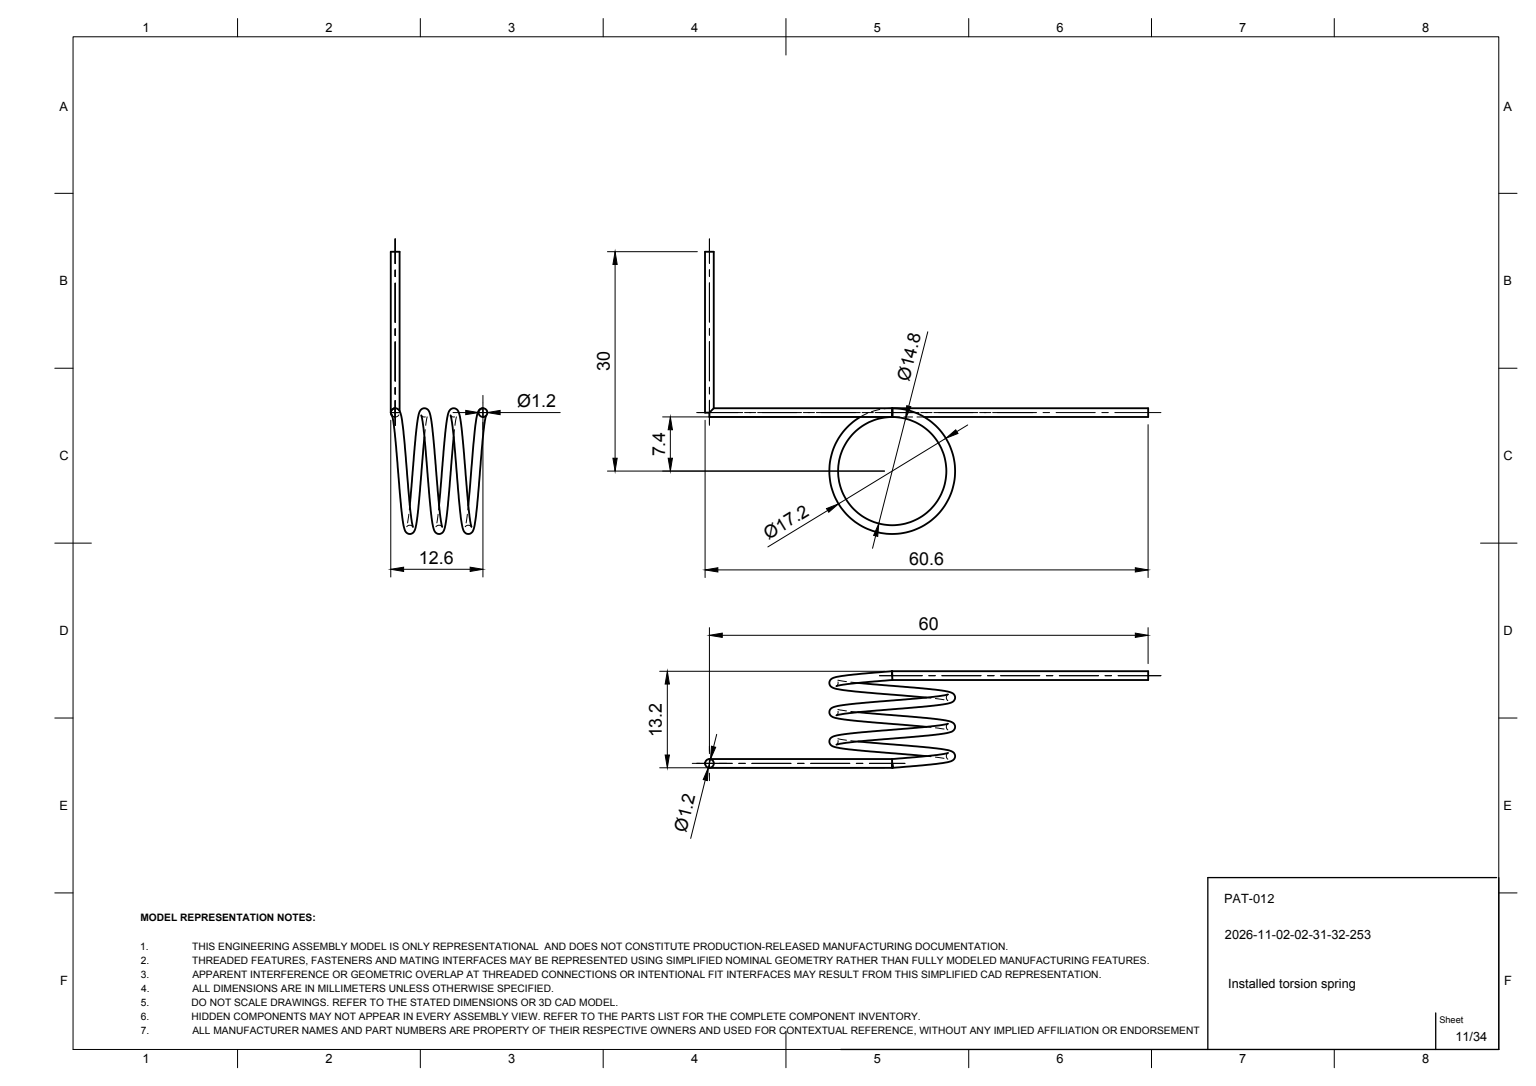
ISO-10303-21;
HEADER;
/* Generated by software containing ST-Developer
 * from STEP Tools, Inc. (www.steptools.com) 
 */

FILE_DESCRIPTION(
/* description */ ('Belt tensioner idler arm'),
/* implementation_level */ '2;1');

FILE_NAME(
/* name */ 'Installed torsion spring.step',
/* time_stamp */ '2026-10-28T03:22:15-07:00',
/* author */ (''),
/* organization */ (''),
/* preprocessor_version */ 'ST-DEVELOPER v20.2',
/* originating_system */ 'Autodesk Translation Framework v15.17.0.0',
/* authorisation */ '');

FILE_SCHEMA (('AUTOMOTIVE_DESIGN { 1 0 10303 214 3 1 1 }'));
ENDSEC;

DATA;
#10=MECHANICAL_DESIGN_GEOMETRIC_PRESENTATION_REPRESENTATION('',(#453),#12779);
#315=B_SPLINE_SURFACE_WITH_KNOTS('',3,3,((#9880,#9881,#9882,#9883,#9884,
#9885,#9886,#9887,#9888,#9889,#9890,#9891,#9892,#9893,#9894,#9895,#9896,
#9897,#9898,#9899,#9900,#9901,#9902,#9903,#9904,#9905,#9906,#9907,#9908,
#9909,#9910,#9911,#9912,#9913,#9914,#9915,#9916,#9917,#9918,#9919,#9920),
(#9921,#9922,#9923,#9924,#9925,#9926,#9927,#9928,#9929,#9930,#9931,#9932,
#9933,#9934,#9935,#9936,#9937,#9938,#9939,#9940,#9941,#9942,#9943,#9944,
#9945,#9946,#9947,#9948,#9949,#9950,#9951,#9952,#9953,#9954,#9955,#9956,
#9957,#9958,#9959,#9960,#9961),(#9962,#9963,#9964,#9965,#9966,#9967,#9968,
#9969,#9970,#9971,#9972,#9973,#9974,#9975,#9976,#9977,#9978,#9979,#9980,
#9981,#9982,#9983,#9984,#9985,#9986,#9987,#9988,#9989,#9990,#9991,#9992,
#9993,#9994,#9995,#9996,#9997,#9998,#9999,#10000,#10001,#10002),(#10003,
#10004,#10005,#10006,#10007,#10008,#10009,#10010,#10011,#10012,#10013,#10014,
#10015,#10016,#10017,#10018,#10019,#10020,#10021,#10022,#10023,#10024,#10025,
#10026,#10027,#10028,#10029,#10030,#10031,#10032,#10033,#10034,#10035,#10036,
#10037,#10038,#10039,#10040,#10041,#10042,#10043),(#10044,#10045,#10046,
#10047,#10048,#10049,#10050,#10051,#10052,#10053,#10054,#10055,#10056,#10057,
#10058,#10059,#10060,#10061,#10062,#10063,#10064,#10065,#10066,#10067,#10068,
#10069,#10070,#10071,#10072,#10073,#10074,#10075,#10076,#10077,#10078,#10079,
#10080,#10081,#10082,#10083,#10084),(#10085,#10086,#10087,#10088,#10089,
#10090,#10091,#10092,#10093,#10094,#10095,#10096,#10097,#10098,#10099,#10100,
#10101,#10102,#10103,#10104,#10105,#10106,#10107,#10108,#10109,#10110,#10111,
#10112,#10113,#10114,#10115,#10116,#10117,#10118,#10119,#10120,#10121,#10122,
#10123,#10124,#10125),(#10126,#10127,#10128,#10129,#10130,#10131,#10132,
#10133,#10134,#10135,#10136,#10137,#10138,#10139,#10140,#10141,#10142,#10143,
#10144,#10145,#10146,#10147,#10148,#10149,#10150,#10151,#10152,#10153,#10154,
#10155,#10156,#10157,#10158,#10159,#10160,#10161,#10162,#10163,#10164,#10165,
#10166),(#10167,#10168,#10169,#10170,#10171,#10172,#10173,#10174,#10175,
#10176,#10177,#10178,#10179,#10180,#10181,#10182,#10183,#10184,#10185,#10186,
#10187,#10188,#10189,#10190,#10191,#10192,#10193,#10194,#10195,#10196,#10197,
#10198,#10199,#10200,#10201,#10202,#10203,#10204,#10205,#10206,#10207),
(#10208,#10209,#10210,#10211,#10212,#10213,#10214,#10215,#10216,#10217,
#10218,#10219,#10220,#10221,#10222,#10223,#10224,#10225,#10226,#10227,#10228,
#10229,#10230,#10231,#10232,#10233,#10234,#10235,#10236,#10237,#10238,#10239,
#10240,#10241,#10242,#10243,#10244,#10245,#10246,#10247,#10248),(#10249,
#10250,#10251,#10252,#10253,#10254,#10255,#10256,#10257,#10258,#10259,#10260,
#10261,#10262,#10263,#10264,#10265,#10266,#10267,#10268,#10269,#10270,#10271,
#10272,#10273,#10274,#10275,#10276,#10277,#10278,#10279,#10280,#10281,#10282,
#10283,#10284,#10285,#10286,#10287,#10288,#10289)),.UNSPECIFIED.,.T.,.F.,
 .F.,(4,1,1,1,1,1,1,4),(4,1,1,1,1,1,1,1,1,1,1,1,1,1,1,1,1,1,1,1,1,1,1,1,
1,1,1,1,1,1,1,1,1,1,1,1,1,1,4),(-3.14159265358988,-2.24399475256421,-1.34639685153853,
-0.448798950512863,0.448798950512809,1.34639685153848,2.24399475256415,
3.14159265358982),(0.,0.0357142857142857,0.0714285714285714,0.107142857142857,
0.125,0.133928571428571,0.142857142857143,0.174603174603175,0.19047619047619,
0.214285714285714,0.238095238095238,0.261904761904762,0.273809523809524,
0.285714285714286,0.30952380952381,0.333333333333333,0.357142857142857,
0.380952380952381,0.412698412698413,0.428571428571429,0.452380952380952,
0.476190476190476,0.5,0.535714285714286,0.571428571428571,0.607142857142857,
0.642857142857143,0.678571428571428,0.714285714285714,0.738095238095238,
0.761904761904762,0.785714285714286,0.809523809523809,0.833333333333333,
0.857142857142857,0.892857142857143,0.928571428571429,0.964285714285714,
1.),.UNSPECIFIED.);
#316=ELLIPSE('',#6695,0.0848528137423855,0.0599999999999996);
#324=B_SPLINE_CURVE_WITH_KNOTS('',3,(#9810,#9811,#9812,#9813,#9814,#9815,
#9816),.UNSPECIFIED.,.F.,.F.,(4,3,4),(-0.00330054689312876,0.,0.00113632995669113),
 .UNSPECIFIED.);
#325=B_SPLINE_CURVE_WITH_KNOTS('',3,(#9817,#9818,#9819,#9820,#9821,#9822,
#9823,#9824,#9825,#9826,#9827,#9828,#9829,#9830,#9831,#9832,#9833,#9834,
#9835,#9836,#9837,#9838,#9839,#9840,#9841,#9842,#9843,#9844,#9845,#9846,
#9847,#9848,#9849,#9850,#9851,#9852,#9853,#9854,#9855,#9856,#9857,#9858,
#9859,#9860,#9861,#9862,#9863,#9864,#9865,#9866,#9867,#9868,#9869,#9870,
#9871,#9872,#9873,#9874),.UNSPECIFIED.,.F.,.F.,(4,3,3,3,3,3,3,3,3,3,3,3,
3,3,3,3,3,3,3,4),(-0.187914936482157,-0.186780639062755,-0.170605853942537,
-0.165437814146277,-0.164113083876462,-0.147906084064185,-0.140662734614346,
-0.124376338567638,-0.117231977811975,-0.111403976662175,-0.095176489596115,
-0.0938100295088016,-0.0774833765802454,-0.070381765801811,-0.0573630234982956,
-0.046936415200375,-0.0306169940923779,-0.0234729466450609,-0.00725345698800663,
-0.00330054689312876),.UNSPECIFIED.);
#326=B_SPLINE_CURVE_WITH_KNOTS('',3,(#10292,#10293,#10294,#10295,#10296,
#10297,#10298,#10299,#10300,#10301,#10302,#10303,#10304,#10305,#10306,#10307,
#10308,#10309,#10310,#10311,#10312,#10313,#10314,#10315,#10316,#10317,#10318,
#10319,#10320,#10321,#10322,#10323,#10324,#10325,#10326,#10327,#10328,#10329,
#10330,#10331,#10332,#10333,#10334,#10335,#10336,#10337,#10338,#10339,#10340,
#10341,#10342,#10343,#10344,#10345,#10346,#10347,#10348,#10349,#10350,#10351,
#10352),.UNSPECIFIED.,.F.,.F.,(4,3,3,3,3,3,3,3,3,3,3,3,3,3,3,3,3,3,3,3,
4),(-0.187914936422243,-0.186780639028976,-0.174403055129874,-0.164113083856377,
-0.147782436669538,-0.140662734596942,-0.124476652868443,-0.120351214576537,
-0.117231977796532,-0.101004644530292,-0.0938100294949805,-0.0775453096070019,
-0.0703817657897228,-0.0663337540103528,-0.0501165597360029,-0.0469364151905663,
-0.0306116886006247,-0.0234729466383474,-0.0122741858231731,0.,0.00113632996403919),
 .UNSPECIFIED.);
#327=B_SPLINE_CURVE_WITH_KNOTS('',3,(#10356,#10357,#10358,#10359,#10360,
#10361,#10362,#10363,#10364,#10365,#10366,#10367,#10368,#10369,#10370,#10371,
#10372,#10373,#10374,#10375,#10376,#10377,#10378,#10379,#10380,#10381,#10382,
#10383,#10384,#10385,#10386,#10387,#10388,#10389,#10390,#10391,#10392,#10393,
#10394,#10395,#10396),.UNSPECIFIED.,.F.,.F.,(4,1,1,1,1,1,1,1,1,1,1,1,1,
1,1,1,1,1,1,1,1,1,1,1,1,1,1,1,1,1,1,1,1,1,1,1,1,1,4),(0.,0.0357142857142857,
0.0714285714285714,0.107142857142857,0.125,0.133928571428571,0.142857142857143,
0.174603174603175,0.19047619047619,0.214285714285714,0.238095238095238,
0.261904761904762,0.273809523809524,0.285714285714286,0.30952380952381,
0.333333333333333,0.357142857142857,0.380952380952381,0.412698412698413,
0.428571428571429,0.452380952380952,0.476190476190476,0.5,0.535714285714286,
0.571428571428571,0.607142857142857,0.642857142857143,0.678571428571428,
0.714285714285714,0.738095238095238,0.761904761904762,0.785714285714286,
0.809523809523809,0.833333333333333,0.857142857142857,0.892857142857143,
0.928571428571429,0.964285714285714,0.999978445633173),.UNSPECIFIED.);
#328=B_SPLINE_CURVE_WITH_KNOTS('',3,(#10397,#10398,#10399,#10400),
 .UNSPECIFIED.,.F.,.F.,(4,4),(0.999978445544819,0.999989048312129),
 .UNSPECIFIED.);
#385=SHAPE_REPRESENTATION_RELATIONSHIP('SRR','None',#12931,#419);
#419=ADVANCED_BREP_SHAPE_REPRESENTATION('',(#495),#12748);
#453=STYLED_ITEM('',(#13184),#495);
#495=MANIFOLD_SOLID_BREP('Body1',#6187);
#693=PLANE('',#6697);
#694=PLANE('',#6698);
#695=PLANE('',#6699);
#696=PLANE('',#6704);
#697=PLANE('',#6705);
#698=PLANE('',#6712);
#699=PLANE('',#6713);
#700=PLANE('',#6714);
#885=FACE_OUTER_BOUND('',#1278,.T.);
#886=FACE_OUTER_BOUND('',#1279,.T.);
#887=FACE_OUTER_BOUND('',#1280,.T.);
#888=FACE_OUTER_BOUND('',#1281,.T.);
#889=FACE_OUTER_BOUND('',#1282,.T.);
#890=FACE_OUTER_BOUND('',#1283,.T.);
#891=FACE_OUTER_BOUND('',#1284,.T.);
#892=FACE_OUTER_BOUND('',#1285,.T.);
#893=FACE_OUTER_BOUND('',#1286,.T.);
#894=FACE_OUTER_BOUND('',#1287,.T.);
#895=FACE_OUTER_BOUND('',#1288,.T.);
#896=FACE_OUTER_BOUND('',#1289,.T.);
#1278=EDGE_LOOP('',(#4280,#4281,#4282,#4283,#4284));
#1279=EDGE_LOOP('',(#4285));
#1280=EDGE_LOOP('',(#4286,#4287));
#1281=EDGE_LOOP('',(#4288,#4289,#4290));
#1282=EDGE_LOOP('',(#4291,#4292,#4293,#4294,#4295,#4296,#4297,#4298));
#1283=EDGE_LOOP('',(#4299,#4300));
#1284=EDGE_LOOP('',(#4301,#4302));
#1285=EDGE_LOOP('',(#4303,#4304,#4305,#4306,#4307,#4308,#4309,#4310,#4311,
#4312));
#1286=EDGE_LOOP('',(#4313,#4314,#4315,#4316,#4317));
#1287=EDGE_LOOP('',(#4318,#4319));
#1288=EDGE_LOOP('',(#4320));
#1289=EDGE_LOOP('',(#4321,#4322,#4323));
#1763=LINE('',#9794,#2112);
#1764=LINE('',#9800,#2113);
#1765=LINE('',#9875,#2114);
#1766=LINE('',#9877,#2115);
#1767=LINE('',#10405,#2116);
#1768=LINE('',#10408,#2117);
#2112=VECTOR('',#7675,0.0599999999999996);
#2113=VECTOR('',#7684,1.);
#2114=VECTOR('',#7695,0.0600000000000001);
#2115=VECTOR('',#7698,1.);
#2116=VECTOR('',#7711,0.06);
#2117=VECTOR('',#7716,1.);
#2439=CIRCLE('',#6694,0.0599999999999996);
#2440=CIRCLE('',#6696,0.0599999999999996);
#2441=CIRCLE('',#6700,0.0600000000000001);
#2442=CIRCLE('',#6701,0.0600000000000001);
#2443=CIRCLE('',#6703,0.0600000000000001);
#2444=CIRCLE('',#6706,0.06);
#2445=CIRCLE('',#6707,0.06);
#2446=CIRCLE('',#6708,0.06);
#2447=CIRCLE('',#6710,0.0600000000000001);
#2448=CIRCLE('',#6711,0.0600000000000001);
#2834=VERTEX_POINT('',#9791);
#2835=VERTEX_POINT('',#9793);
#2836=VERTEX_POINT('',#9795);
#2837=VERTEX_POINT('',#9802);
#2838=VERTEX_POINT('',#9806);
#2839=VERTEX_POINT('',#9807);
#2840=VERTEX_POINT('',#9809);
#2841=VERTEX_POINT('',#10290);
#2842=VERTEX_POINT('',#10291);
#2843=VERTEX_POINT('',#10353);
#2844=VERTEX_POINT('',#10355);
#2845=VERTEX_POINT('',#10404);
#3395=EDGE_CURVE('',#2834,#2834,#2439,.T.);
#3396=EDGE_CURVE('',#2834,#2835,#1763,.T.);
#3397=EDGE_CURVE('',#2836,#2835,#316,.T.);
#3398=EDGE_CURVE('',#2836,#2835,#2440,.T.);
#3399=EDGE_CURVE('',#2835,#2836,#1764,.T.);
#3400=EDGE_CURVE('',#2836,#2837,#2441,.T.);
#3401=EDGE_CURVE('',#2837,#2835,#2442,.T.);
#3402=EDGE_CURVE('',#2838,#2839,#2443,.T.);
#3403=EDGE_CURVE('',#2840,#2839,#324,.T.);
#3404=EDGE_CURVE('',#2838,#2840,#325,.T.);
#3405=EDGE_CURVE('',#2837,#2838,#1765,.T.);
#3406=EDGE_CURVE('',#2839,#2838,#1766,.T.);
#3407=EDGE_CURVE('',#2838,#2839,#2444,.T.);
#3408=EDGE_CURVE('',#2841,#2842,#326,.T.);
#3409=EDGE_CURVE('',#2842,#2843,#2445,.T.);
#3410=EDGE_CURVE('',#2843,#2844,#327,.T.);
#3411=EDGE_CURVE('',#2844,#2840,#328,.T.);
#3412=EDGE_CURVE('',#2843,#2841,#2446,.T.);
#3413=EDGE_CURVE('',#2842,#2841,#2447,.T.);
#3414=EDGE_CURVE('',#2841,#2845,#1767,.T.);
#3415=EDGE_CURVE('',#2845,#2845,#2448,.T.);
#3416=EDGE_CURVE('',#2842,#2841,#1768,.T.);
#4280=ORIENTED_EDGE('',*,*,#3395,.F.);
#4281=ORIENTED_EDGE('',*,*,#3396,.T.);
#4282=ORIENTED_EDGE('',*,*,#3397,.F.);
#4283=ORIENTED_EDGE('',*,*,#3398,.T.);
#4284=ORIENTED_EDGE('',*,*,#3396,.F.);
#4285=ORIENTED_EDGE('',*,*,#3395,.T.);
#4286=ORIENTED_EDGE('',*,*,#3399,.F.);
#4287=ORIENTED_EDGE('',*,*,#3398,.F.);
#4288=ORIENTED_EDGE('',*,*,#3399,.T.);
#4289=ORIENTED_EDGE('',*,*,#3400,.T.);
#4290=ORIENTED_EDGE('',*,*,#3401,.T.);
#4291=ORIENTED_EDGE('',*,*,#3402,.T.);
#4292=ORIENTED_EDGE('',*,*,#3403,.F.);
#4293=ORIENTED_EDGE('',*,*,#3404,.F.);
#4294=ORIENTED_EDGE('',*,*,#3405,.F.);
#4295=ORIENTED_EDGE('',*,*,#3400,.F.);
#4296=ORIENTED_EDGE('',*,*,#3397,.T.);
#4297=ORIENTED_EDGE('',*,*,#3401,.F.);
#4298=ORIENTED_EDGE('',*,*,#3405,.T.);
#4299=ORIENTED_EDGE('',*,*,#3406,.F.);
#4300=ORIENTED_EDGE('',*,*,#3402,.F.);
#4301=ORIENTED_EDGE('',*,*,#3406,.T.);
#4302=ORIENTED_EDGE('',*,*,#3407,.T.);
#4303=ORIENTED_EDGE('',*,*,#3408,.T.);
#4304=ORIENTED_EDGE('',*,*,#3409,.T.);
#4305=ORIENTED_EDGE('',*,*,#3410,.T.);
#4306=ORIENTED_EDGE('',*,*,#3411,.T.);
#4307=ORIENTED_EDGE('',*,*,#3403,.T.);
#4308=ORIENTED_EDGE('',*,*,#3407,.F.);
#4309=ORIENTED_EDGE('',*,*,#3404,.T.);
#4310=ORIENTED_EDGE('',*,*,#3411,.F.);
#4311=ORIENTED_EDGE('',*,*,#3410,.F.);
#4312=ORIENTED_EDGE('',*,*,#3412,.T.);
#4313=ORIENTED_EDGE('',*,*,#3413,.F.);
#4314=ORIENTED_EDGE('',*,*,#3408,.F.);
#4315=ORIENTED_EDGE('',*,*,#3414,.T.);
#4316=ORIENTED_EDGE('',*,*,#3415,.T.);
#4317=ORIENTED_EDGE('',*,*,#3414,.F.);
#4318=ORIENTED_EDGE('',*,*,#3416,.F.);
#4319=ORIENTED_EDGE('',*,*,#3413,.T.);
#4320=ORIENTED_EDGE('',*,*,#3415,.F.);
#4321=ORIENTED_EDGE('',*,*,#3416,.T.);
#4322=ORIENTED_EDGE('',*,*,#3412,.F.);
#4323=ORIENTED_EDGE('',*,*,#3409,.F.);
#5680=CYLINDRICAL_SURFACE('',#6693,0.0599999999999996);
#5681=CYLINDRICAL_SURFACE('',#6702,0.0600000000000001);
#5682=CYLINDRICAL_SURFACE('',#6709,0.0600000000000001);
#5862=ADVANCED_FACE('',(#885),#5680,.T.);
#5863=ADVANCED_FACE('',(#886),#693,.T.);
#5864=ADVANCED_FACE('',(#887),#694,.F.);
#5865=ADVANCED_FACE('',(#888),#695,.T.);
#5866=ADVANCED_FACE('',(#889),#5681,.T.);
#5867=ADVANCED_FACE('',(#890),#696,.F.);
#5868=ADVANCED_FACE('',(#891),#697,.T.);
#5869=ADVANCED_FACE('',(#892),#315,.T.);
#5870=ADVANCED_FACE('',(#893),#5682,.T.);
#5871=ADVANCED_FACE('',(#894),#698,.T.);
#5872=ADVANCED_FACE('',(#895),#699,.F.);
#5873=ADVANCED_FACE('',(#896),#700,.F.);
#6187=CLOSED_SHELL('',(#5862,#5863,#5864,#5865,#5866,#5867,#5868,#5869,
#5870,#5871,#5872,#5873));
#6692=AXIS2_PLACEMENT_3D('',#9789,#7669,#7670);
#6693=AXIS2_PLACEMENT_3D('',#9790,#7671,#7672);
#6694=AXIS2_PLACEMENT_3D('',#9792,#7673,#7674);
#6695=AXIS2_PLACEMENT_3D('',#9796,#7676,#7677);
#6696=AXIS2_PLACEMENT_3D('',#9797,#7678,#7679);
#6697=AXIS2_PLACEMENT_3D('',#9798,#7680,#7681);
#6698=AXIS2_PLACEMENT_3D('',#9799,#7682,#7683);
#6699=AXIS2_PLACEMENT_3D('',#9801,#7685,#7686);
#6700=AXIS2_PLACEMENT_3D('',#9803,#7687,#7688);
#6701=AXIS2_PLACEMENT_3D('',#9804,#7689,#7690);
#6702=AXIS2_PLACEMENT_3D('',#9805,#7691,#7692);
#6703=AXIS2_PLACEMENT_3D('',#9808,#7693,#7694);
#6704=AXIS2_PLACEMENT_3D('',#9876,#7696,#7697);
#6705=AXIS2_PLACEMENT_3D('',#9878,#7699,#7700);
#6706=AXIS2_PLACEMENT_3D('',#9879,#7701,#7702);
#6707=AXIS2_PLACEMENT_3D('',#10354,#7703,#7704);
#6708=AXIS2_PLACEMENT_3D('',#10401,#7705,#7706);
#6709=AXIS2_PLACEMENT_3D('',#10402,#7707,#7708);
#6710=AXIS2_PLACEMENT_3D('',#10403,#7709,#7710);
#6711=AXIS2_PLACEMENT_3D('',#10406,#7712,#7713);
#6712=AXIS2_PLACEMENT_3D('',#10407,#7714,#7715);
#6713=AXIS2_PLACEMENT_3D('',#10409,#7717,#7718);
#6714=AXIS2_PLACEMENT_3D('',#10410,#7719,#7720);
#7669=DIRECTION('axis',(0.,0.,1.));
#7670=DIRECTION('refdir',(1.,0.,0.));
#7671=DIRECTION('center_axis',(1.,0.,0.));
#7672=DIRECTION('ref_axis',(0.,0.,-1.));
#7673=DIRECTION('center_axis',(1.,0.,0.));
#7674=DIRECTION('ref_axis',(0.,0.,-1.));
#7675=DIRECTION('',(-1.,0.,0.));
#7676=DIRECTION('center_axis',(-0.707106781186545,-0.70710678118655,0.));
#7677=DIRECTION('ref_axis',(-0.70710678118655,0.707106781186545,0.));
#7678=DIRECTION('center_axis',(1.,0.,0.));
#7679=DIRECTION('ref_axis',(0.,0.,-1.));
#7680=DIRECTION('center_axis',(1.,0.,0.));
#7681=DIRECTION('ref_axis',(0.,0.,-1.));
#7682=DIRECTION('center_axis',(1.,0.,0.));
#7683=DIRECTION('ref_axis',(0.,0.,-1.));
#7684=DIRECTION('',(0.,0.,-1.));
#7685=DIRECTION('center_axis',(0.,1.,0.));
#7686=DIRECTION('ref_axis',(1.,0.,0.));
#7687=DIRECTION('center_axis',(0.,1.,0.));
#7688=DIRECTION('ref_axis',(1.,0.,0.));
#7689=DIRECTION('center_axis',(0.,1.,0.));
#7690=DIRECTION('ref_axis',(1.,0.,0.));
#7691=DIRECTION('center_axis',(0.,1.,0.));
#7692=DIRECTION('ref_axis',(1.,0.,0.));
#7693=DIRECTION('center_axis',(0.,1.,0.));
#7694=DIRECTION('ref_axis',(1.,0.,0.));
#7695=DIRECTION('',(0.,-1.,0.));
#7696=DIRECTION('center_axis',(0.,1.,0.));
#7697=DIRECTION('ref_axis',(1.,0.,0.));
#7698=DIRECTION('',(-0.999998524452206,0.,0.00171787467842657));
#7699=DIRECTION('center_axis',(0.000135869566583555,0.996867347600064,0.0790915471354176));
#7700=DIRECTION('ref_axis',(-0.997148648532913,-0.00583337009538651,0.0752365903155829));
#7701=DIRECTION('center_axis',(0.000135869566583555,0.996867347600064,0.0790915471354176));
#7702=DIRECTION('ref_axis',(-0.997148648532913,-0.00583337009538652,0.0752365903155829));
#7703=DIRECTION('center_axis',(-0.000135869608553456,0.996867347637577,
0.0790915466625346));
#7704=DIRECTION('ref_axis',(1.07799070862851E-5,-0.0790915459279024,0.996867356896858));
#7705=DIRECTION('center_axis',(-0.000135869608553456,0.996867347637577,
0.0790915466625346));
#7706=DIRECTION('ref_axis',(1.07799070862851E-5,-0.0790915459279024,0.996867356896858));
#7707=DIRECTION('center_axis',(0.,1.,0.));
#7708=DIRECTION('ref_axis',(1.,0.,0.));
#7709=DIRECTION('center_axis',(0.,1.,0.));
#7710=DIRECTION('ref_axis',(1.,0.,0.));
#7711=DIRECTION('',(0.,-1.,0.));
#7712=DIRECTION('center_axis',(0.,1.,0.));
#7713=DIRECTION('ref_axis',(1.,0.,0.));
#7714=DIRECTION('center_axis',(0.,1.,0.));
#7715=DIRECTION('ref_axis',(1.,0.,0.));
#7716=DIRECTION('',(-0.999998524451277,0.,-0.0017178752193449));
#7717=DIRECTION('center_axis',(0.,1.,0.));
#7718=DIRECTION('ref_axis',(1.,0.,0.));
#7719=DIRECTION('center_axis',(-0.000135869608553456,0.996867347637577,
0.0790915466625346));
#7720=DIRECTION('ref_axis',(1.07799070862851E-5,-0.0790915459279024,0.996867356896858));
#9789=CARTESIAN_POINT('',(0.,0.,0.));
#9790=CARTESIAN_POINT('Origin',(0.8,2.5,8.05));
#9791=CARTESIAN_POINT('',(3.,2.5,8.11));
#9792=CARTESIAN_POINT('Origin',(3.,2.5,8.05));
#9793=CARTESIAN_POINT('',(0.8,2.5,8.11));
#9794=CARTESIAN_POINT('',(0.8,2.5,8.11));
#9795=CARTESIAN_POINT('',(0.8,2.5,7.99));
#9796=CARTESIAN_POINT('Origin',(0.8,2.5,8.05));
#9797=CARTESIAN_POINT('Origin',(0.8,2.5,8.05));
#9798=CARTESIAN_POINT('Origin',(3.,2.5,8.05));
#9799=CARTESIAN_POINT('Origin',(0.8,2.5,8.05));
#9800=CARTESIAN_POINT('',(0.8,2.5,8.05));
#9801=CARTESIAN_POINT('Origin',(0.8,2.5,8.05));
#9802=CARTESIAN_POINT('',(0.74,2.5,8.05));
#9803=CARTESIAN_POINT('Origin',(0.8,2.5,8.05));
#9804=CARTESIAN_POINT('Origin',(0.8,2.5,8.05));
#9805=CARTESIAN_POINT('Origin',(0.8,0.,8.05));
#9806=CARTESIAN_POINT('',(0.740018061544387,3.68116671391522E-6,8.05003232801258));
#9807=CARTESIAN_POINT('',(0.859999911467134,-6.70801305127644E-14,8.04989692752013));
#9808=CARTESIAN_POINT('Origin',(0.8,0.,8.05));
#9809=CARTESIAN_POINT('',(0.859872085377142,0.000172980010645474,8.04546127555641));
#9810=CARTESIAN_POINT('Ctrl Pts',(0.859872085377143,0.000172980010644996,
8.04546127555642));
#9811=CARTESIAN_POINT('Ctrl Pts',(0.859954613291757,0.00013063375777587,
8.04655234991555));
#9812=CARTESIAN_POINT('Ctrl Pts',(0.860005150486507,8.81606608541971E-5,
8.04764678325301));
#9813=CARTESIAN_POINT('Ctrl Pts',(0.860024122218985,4.56008323849017E-5,
8.0487434141295));
#9814=CARTESIAN_POINT('Ctrl Pts',(0.860030653976549,3.0947954381455E-5,
8.04912097200569));
#9815=CARTESIAN_POINT('Ctrl Pts',(0.860033440268576,1.62917027234746E-5,
8.04949861025168));
#9816=CARTESIAN_POINT('Ctrl Pts',(0.86003250673194,1.63365101006011E-6,
8.0498762810392));
#9817=CARTESIAN_POINT('Ctrl Pts',(0.740037512403726,7.66502084125951E-6,
8.04995576651375));
#9818=CARTESIAN_POINT('Ctrl Pts',(0.740035813633067,2.29745219354216E-5,
8.04957722865058));
#9819=CARTESIAN_POINT('Ctrl Pts',(0.740037570114014,3.82814117523058E-5,
8.04919872536356));
#9820=CARTESIAN_POINT('Ctrl Pts',(0.740042788070948,5.3583348281363E-5,
8.04882030923245));
#9821=CARTESIAN_POINT('Ctrl Pts',(0.740117194774797,0.000271784968983559,
8.04342419397895));
#9822=CARTESIAN_POINT('Ctrl Pts',(0.740890792150363,0.000487598405839051,
8.03808128898406));
#9823=CARTESIAN_POINT('Ctrl Pts',(0.742380657699473,0.000694100304033197,
8.03294245997655));
#9824=CARTESIAN_POINT('Ctrl Pts',(0.742856687791474,0.000760080162185162,
8.03130054185402));
#9825=CARTESIAN_POINT('Ctrl Pts',(0.743406227546339,0.000825107328953121,
8.02967950161156));
#9826=CARTESIAN_POINT('Ctrl Pts',(0.744030943387962,0.000888935459998242,
8.02808458212714));
#9827=CARTESIAN_POINT('Ctrl Pts',(0.744191077600943,0.000905296606698836,
8.02767575436996));
#9828=CARTESIAN_POINT('Ctrl Pts',(0.744356154182508,0.000921578861224115,
8.02726864444978));
#9829=CARTESIAN_POINT('Ctrl Pts',(0.744526114805664,0.000937780810410216,
8.02686330823041));
#9830=CARTESIAN_POINT('Ctrl Pts',(0.746605445104324,0.00113599851057101,
8.02190434852298));
#9831=CARTESIAN_POINT('Ctrl Pts',(0.749384937540555,0.00131981950420992,
8.01727240895181));
#9832=CARTESIAN_POINT('Ctrl Pts',(0.752732134934782,0.00148661196187375,
8.01305741080169));
#9833=CARTESIAN_POINT('Ctrl Pts',(0.754228088577332,0.00156115605210947,
8.01117361337555));
#9834=CARTESIAN_POINT('Ctrl Pts',(0.755838113800148,0.00163228884922257,
8.00937339005261));
#9835=CARTESIAN_POINT('Ctrl Pts',(0.757553006477384,0.00169967923105377,
8.0076667868923));
#9836=CARTESIAN_POINT('Ctrl Pts',(0.761408877509493,0.00185120394428867,
8.00382955452406));
#9837=CARTESIAN_POINT('Ctrl Pts',(0.765741812850314,0.00198196807366009,
8.00051359678304));
#9838=CARTESIAN_POINT('Ctrl Pts',(0.770433984217127,0.00208730979332829,
7.99782013360317));
#9839=CARTESIAN_POINT('Ctrl Pts',(0.772492301163109,0.00213352009337093,
7.99663859088593));
#9840=CARTESIAN_POINT('Ctrl Pts',(0.774620207181123,0.00217481038890225,
7.99557731561769));
#9841=CARTESIAN_POINT('Ctrl Pts',(0.776809296807154,0.00221060862651016,
7.99464766697112));
#9842=CARTESIAN_POINT('Ctrl Pts',(0.778595043257235,0.00223981098303675,
7.99388930753682));
#9843=CARTESIAN_POINT('Ctrl Pts',(0.78041309647326,0.00226521029907004,
7.99322216165319));
#9844=CARTESIAN_POINT('Ctrl Pts',(0.782258231705198,0.00228650951969933,
7.99265080830793));
#9845=CARTESIAN_POINT('Ctrl Pts',(0.787395826455402,0.00234581507204828,
7.99105993198825));
#9846=CARTESIAN_POINT('Ctrl Pts',(0.79274285347778,0.00237362730590223,
7.99020783651138));
#9847=CARTESIAN_POINT('Ctrl Pts',(0.798148945965851,0.00237405188957915,
7.99006491773579));
#9848=CARTESIAN_POINT('Ctrl Pts',(0.798604174158806,0.00237408764228971,
7.99005288304418));
#9849=CARTESIAN_POINT('Ctrl Pts',(0.799059822737112,0.00237392689538011,
7.99004590715478));
#9850=CARTESIAN_POINT('Ctrl Pts',(0.799515801280592,0.00237357083570519,
7.99004398888629));
#9851=CARTESIAN_POINT('Ctrl Pts',(0.804963895587468,0.00236931658577196,
7.99002106915075));
#9852=CARTESIAN_POINT('Ctrl Pts',(0.810387077449856,0.00233753275049762,
7.99071609996183));
#9853=CARTESIAN_POINT('Ctrl Pts',(0.815632511887815,0.00228013906244369,
7.99209871900176));
#9854=CARTESIAN_POINT('Ctrl Pts',(0.817914120610998,0.002255174506911,7.99270011736059));
#9855=CARTESIAN_POINT('Ctrl Pts',(0.820162094552721,0.00222530653908412,
7.99343227420397));
#9856=CARTESIAN_POINT('Ctrl Pts',(0.822363029819604,0.002190429374402,7.99429566671149));
#9857=CARTESIAN_POINT('Ctrl Pts',(0.82639780586693,0.00212649221515163,
7.99587844629669));
#9858=CARTESIAN_POINT('Ctrl Pts',(0.830232389001066,0.0020464716033856,
7.99788444042298));
#9859=CARTESIAN_POINT('Ctrl Pts',(0.833789300856325,0.00194967646796662,
8.00030488653809));
#9860=CARTESIAN_POINT('Ctrl Pts',(0.836638003580475,0.00187215400545616,
8.00224340279105));
#9861=CARTESIAN_POINT('Ctrl Pts',(0.839308650131527,0.00178382077303799,
8.00444829662651));
#9862=CARTESIAN_POINT('Ctrl Pts',(0.841781595032497,0.00168657107783632,
8.00688404387467));
#9863=CARTESIAN_POINT('Ctrl Pts',(0.845652175768119,0.00153435871085521,
8.0106964039365));
#9864=CARTESIAN_POINT('Ctrl Pts',(0.848989336192329,0.00136248698922647,
8.01502206971187));
#9865=CARTESIAN_POINT('Ctrl Pts',(0.851727216776977,0.00117766887422212,
8.01971434681324));
#9866=CARTESIAN_POINT('Ctrl Pts',(0.852925761055746,0.00109676224316106,
8.02176845461684));
#9867=CARTESIAN_POINT('Ctrl Pts',(0.854008975753402,0.00101332668916306,
8.02389331395814));
#9868=CARTESIAN_POINT('Ctrl Pts',(0.854968645475949,0.000927759185469039,
8.02607820491659));
#9869=CARTESIAN_POINT('Ctrl Pts',(0.857147435543468,0.000733490654566433,
8.03103868101274));
#9870=CARTESIAN_POINT('Ctrl Pts',(0.858664126628259,0.000530921213849663,
8.03624259871879));
#9871=CARTESIAN_POINT('Ctrl Pts',(0.85943954321166,0.000324530879757094,
8.04155733118659));
#9872=CARTESIAN_POINT('Ctrl Pts',(0.859628522772982,0.000274230749952153,
8.04285260373016));
#9873=CARTESIAN_POINT('Ctrl Pts',(0.859773244368349,0.00022369573125849,
8.04415453107995));
#9874=CARTESIAN_POINT('Ctrl Pts',(0.859872085377142,0.000172980010645474,
8.04546127555641));
#9875=CARTESIAN_POINT('',(0.74,0.,8.05));
#9876=CARTESIAN_POINT('Origin',(0.8,0.,8.05));
#9877=CARTESIAN_POINT('',(0.8,0.,8.04999999999999));
#9878=CARTESIAN_POINT('Origin',(0.8,-6.66133814775094E-16,8.05));
#9879=CARTESIAN_POINT('Origin',(0.8,-6.66133814775094E-16,8.05));
#9880=CARTESIAN_POINT('Ctrl Pts',(0.799992192036797,0.00474896193479852,
6.79014422086044));
#9881=CARTESIAN_POINT('Ctrl Pts',(0.799967638550529,0.184896450338747,6.80443713908974));
#9882=CARTESIAN_POINT('Ctrl Pts',(0.674670361705441,0.543455008309391,6.8330594352144));
#9883=CARTESIAN_POINT('Ctrl Pts',(0.189034209544693,0.849439608053688,6.87617354971506));
#9884=CARTESIAN_POINT('Ctrl Pts',(-0.287258299249701,0.795379885058583,
6.91224027998794));
#9885=CARTESIAN_POINT('Ctrl Pts',(-0.550325497980241,0.607926215999118,
6.93756224237155));
#9886=CARTESIAN_POINT('Ctrl Pts',(-0.668135787638992,0.468370262290034,
6.95205278987894));
#9887=CARTESIAN_POINT('Ctrl Pts',(-0.797681515793003,0.249601245171223,
6.97219797725517));
#9888=CARTESIAN_POINT('Ctrl Pts',(-0.842241289744138,-0.0491002547813337,
6.99521334099182));
#9889=CARTESIAN_POINT('Ctrl Pts',(-0.732812122296168,-0.403197173369283,
7.02435916833342));
#9890=CARTESIAN_POINT('Ctrl Pts',(-0.524668382980495,-0.664806008100517,
7.0503201318013));
#9891=CARTESIAN_POINT('Ctrl Pts',(-0.184652568425117,-0.828760962866216,
7.07959861118036));
#9892=CARTESIAN_POINT('Ctrl Pts',(0.130453782933179,-0.82870656943649,7.10405631433573));
#9893=CARTESIAN_POINT('Ctrl Pts',(0.364375751582702,-0.746687575144636,
7.12365775087804));
#9894=CARTESIAN_POINT('Ctrl Pts',(0.574616121324387,-0.614810215974657,
7.14328235821488));
#9895=CARTESIAN_POINT('Ctrl Pts',(0.772150732123964,-0.367420603086453,
7.16785616546509));
#9896=CARTESIAN_POINT('Ctrl Pts',(0.856997117769862,0.00408861547259015,
7.19741267271575));
#9897=CARTESIAN_POINT('Ctrl Pts',(0.772201652552023,0.376032772307348,7.22703591400899));
#9898=CARTESIAN_POINT('Ctrl Pts',(0.507351873091063,0.709199534687239,7.26002305113266));
#9899=CARTESIAN_POINT('Ctrl Pts',(0.143736848284574,0.852002078379093,7.28978615651597));
#9900=CARTESIAN_POINT('Ctrl Pts',(-0.234502546384647,0.823108658745492,
7.31961111148852));
#9901=CARTESIAN_POINT('Ctrl Pts',(-0.542883282495364,0.675129422402413,
7.34616719094667));
#9902=CARTESIAN_POINT('Ctrl Pts',(-0.783396359273759,0.37345029211527,7.3761020331664));
#9903=CARTESIAN_POINT('Ctrl Pts',(-0.884489493081995,-0.0661466723839558,
7.41109301032321));
#9904=CARTESIAN_POINT('Ctrl Pts',(-0.709418296017906,-0.569369739308696,
7.45117535759087));
#9905=CARTESIAN_POINT('Ctrl Pts',(-0.19989068769657,-0.889667511851702,
7.49638689971083));
#9906=CARTESIAN_POINT('Ctrl Pts',(0.398973895326053,-0.822339305277361,
7.54171055210185));
#9907=CARTESIAN_POINT('Ctrl Pts',(0.826865587387622,-0.395358142551438,
7.58713932258037));
#9908=CARTESIAN_POINT('Ctrl Pts',(0.894293657405342,0.206666783144423,7.6326658525427));
#9909=CARTESIAN_POINT('Ctrl Pts',(0.607352590357856,0.662764035303079,7.67321405418637));
#9910=CARTESIAN_POINT('Ctrl Pts',(0.194215191945802,0.860916697467946,7.70874703376387));
#9911=CARTESIAN_POINT('Ctrl Pts',(-0.198496552114366,0.86128604965953,7.7392380606388));
#9912=CARTESIAN_POINT('Ctrl Pts',(-0.552965374281963,0.690483866395827,
7.76976084505319));
#9913=CARTESIAN_POINT('Ctrl Pts',(-0.798625493103115,0.382774108679761,
7.80031292414605));
#9914=CARTESIAN_POINT('Ctrl Pts',(-0.886090514398701,-0.00135276288038935,
7.83089169974969));
#9915=CARTESIAN_POINT('Ctrl Pts',(-0.784450923473031,-0.450417071001065,
7.86659566812776));
#9916=CARTESIAN_POINT('Ctrl Pts',(-0.401130832210515,-0.834733160113732,
7.90743505712395));
#9917=CARTESIAN_POINT('Ctrl Pts',(0.206987829997999,-0.903462960885791,
7.95342319362056));
#9918=CARTESIAN_POINT('Ctrl Pts',(0.725081242328631,-0.57760276120548,7.99943459556092));
#9919=CARTESIAN_POINT('Ctrl Pts',(0.859845779758374,-0.192969267412252,
8.03013735189051));
#9920=CARTESIAN_POINT('Ctrl Pts',(0.85987212861708,0.000350822954683268,
8.04547538565828));
#9921=CARTESIAN_POINT('Ctrl Pts',(0.782083895515197,0.00474658906385578,
6.7901433641864));
#9922=CARTESIAN_POINT('Ctrl Pts',(0.782059882823066,0.180926302609037,6.804121478795));
#9923=CARTESIAN_POINT('Ctrl Pts',(0.659555973271399,0.531487716947758,6.8321048287837));
#9924=CARTESIAN_POINT('Ctrl Pts',(0.184633116814794,0.830760271314604,6.87426980269771));
#9925=CARTESIAN_POINT('Ctrl Pts',(-0.281260451809225,0.77788801176931,6.90954769821697));
#9926=CARTESIAN_POINT('Ctrl Pts',(-0.538641971540873,0.594493606073614,
6.93432208193731));
#9927=CARTESIAN_POINT('Ctrl Pts',(-0.653918190481005,0.457939407603894,
6.94850083234196));
#9928=CARTESIAN_POINT('Ctrl Pts',(-0.780687953317182,0.24386073084139,6.96821417260151));
#9929=CARTESIAN_POINT('Ctrl Pts',(-0.824314307227793,-0.0484926765471151,
6.99074018142266));
#9930=CARTESIAN_POINT('Ctrl Pts',(-0.717187592119459,-0.39515858636662,
7.01927419391762));
#9931=CARTESIAN_POINT('Ctrl Pts',(-0.513375485381163,-0.651339249880567,
7.04469559652104));
#9932=CARTESIAN_POINT('Ctrl Pts',(-0.18032688172712,-0.811949801148858,
7.07337464673134));
#9933=CARTESIAN_POINT('Ctrl Pts',(0.128427340685738,-0.811907838078087,
7.09733900644489));
#9934=CARTESIAN_POINT('Ctrl Pts',(0.357695972714028,-0.731523164591556,
7.11655037491275));
#9935=CARTESIAN_POINT('Ctrl Pts',(0.563791009551169,-0.602248940512661,
7.13578788095882));
#9936=CARTESIAN_POINT('Ctrl Pts',(0.75749315843225,-0.359680144541225,7.15988348127248));
#9937=CARTESIAN_POINT('Ctrl Pts',(0.840739127744584,0.00474265771027548,
7.18887631751055));
#9938=CARTESIAN_POINT('Ctrl Pts',(0.757542143832615,0.369752074104698,7.21794685951956));
#9939=CARTESIAN_POINT('Ctrl Pts',(0.497538985691502,0.69685828530355,7.25033241461142));
#9940=CARTESIAN_POINT('Ctrl Pts',(0.14037263865275,0.837164983887327,7.27956858898822));
#9941=CARTESIAN_POINT('Ctrl Pts',(-0.23135335299626,0.808779563585517,7.30887964110316));
#9942=CARTESIAN_POINT('Ctrl Pts',(-0.534553583157228,0.663306227172658,
7.33498883247858));
#9943=CARTESIAN_POINT('Ctrl Pts',(-0.771160823931885,0.366562149115926,
7.36443528633921));
#9944=CARTESIAN_POINT('Ctrl Pts',(-0.870684139974891,-0.066085974814,7.39887368559955));
#9945=CARTESIAN_POINT('Ctrl Pts',(-0.698328687945324,-0.561724009713536,
7.43834986568262));
#9946=CARTESIAN_POINT('Ctrl Pts',(-0.196117757216787,-0.877529134736446,
7.48291619387264));
#9947=CARTESIAN_POINT('Ctrl Pts',(0.394743019079569,-0.811191649286449,
7.52763305566212));
#9948=CARTESIAN_POINT('Ctrl Pts',(0.81736602063245,-0.389604577121731,7.57249504917915));
#9949=CARTESIAN_POINT('Ctrl Pts',(0.884116043254209,0.205474962906694,7.61749685897569));
#9950=CARTESIAN_POINT('Ctrl Pts',(0.600276565017539,0.656805803364734,7.65761681609474));
#9951=CARTESIAN_POINT('Ctrl Pts',(0.191169205453925,0.853065704046926,7.69280415993483));
#9952=CARTESIAN_POINT('Ctrl Pts',(-0.19798749521213,0.853460360938559,7.72301919980889));
#9953=CARTESIAN_POINT('Ctrl Pts',(-0.549503313068882,0.68411551039788,7.75328641528884));
#9954=CARTESIAN_POINT('Ctrl Pts',(-0.793301852382218,0.378787453389241,
7.78360396950921));
#9955=CARTESIAN_POINT('Ctrl Pts',(-0.880186024863404,-0.00265264652523096,
7.81396924276319));
#9956=CARTESIAN_POINT('Ctrl Pts',(-0.779222443771506,-0.448904993517531,
7.84944930171758));
#9957=CARTESIAN_POINT('Ctrl Pts',(-0.398034992400597,-0.831218430880183,
7.89006870656519));
#9958=CARTESIAN_POINT('Ctrl Pts',(0.207454027684503,-0.899761502606193,
7.93585934905774));
#9959=CARTESIAN_POINT('Ctrl Pts',(0.723947436484212,-0.575045194343942,
7.98172266468812));
#9960=CARTESIAN_POINT('Ctrl Pts',(0.858495280337168,-0.191231028022566,
8.01236184878027));
#9961=CARTESIAN_POINT('Ctrl Pts',(0.858521584804765,0.00176336728401826,
8.02767404187196));
#9962=CARTESIAN_POINT('Ctrl Pts',(0.746211861175701,0.00337911061953199,
6.80731739539198));
#9963=CARTESIAN_POINT('Ctrl Pts',(0.746188933644134,0.171597064764558,6.82066382328057));
#9964=CARTESIAN_POINT('Ctrl Pts',(0.629300643905895,0.505942199544543,6.84735079201033));
#9965=CARTESIAN_POINT('Ctrl Pts',(0.176589535284547,0.791165596604293,6.88754110635019));
#9966=CARTESIAN_POINT('Ctrl Pts',(-0.267122090093055,0.740741855173879,
6.92113590965913));
#9967=CARTESIAN_POINT('Ctrl Pts',(-0.512154380788647,0.566142234255932,
6.94472155200791));
#9968=CARTESIAN_POINT('Ctrl Pts',(-0.621881987091332,0.43615820692645,6.95821760793587));
#9969=CARTESIAN_POINT('Ctrl Pts',(-0.74253529346074,0.232406920931183,6.97697939452374));
#9970=CARTESIAN_POINT('Ctrl Pts',(-0.784032142894782,-0.0457619996394047,
6.99841041192963));
#9971=CARTESIAN_POINT('Ctrl Pts',(-0.682117732110117,-0.375558705039205,
7.02555581439515));
#9972=CARTESIAN_POINT('Ctrl Pts',(-0.488256756238947,-0.619222960670186,
7.04973308403748));
#9973=CARTESIAN_POINT('Ctrl Pts',(-0.171488008056215,-0.771983305067387,
7.0770099902553));
#9974=CARTESIAN_POINT('Ctrl Pts',(0.122149257398574,-0.771940192929056,
7.09979855320445));
#9975=CARTESIAN_POINT('Ctrl Pts',(0.340211353718798,-0.695486110106044,
7.11807045248607));
#9976=CARTESIAN_POINT('Ctrl Pts',(0.53623820285835,-0.572527321706746,7.13636752838297));
#9977=CARTESIAN_POINT('Ctrl Pts',(0.720489227996175,-0.341802196164832,
7.15928518411744));
#9978=CARTESIAN_POINT('Ctrl Pts',(0.799693173144715,0.00489118347571509,
7.1868659148334));
#9979=CARTESIAN_POINT('Ctrl Pts',(0.720533952481635,0.35223376988072,7.21452830637497));
#9980=CARTESIAN_POINT('Ctrl Pts',(0.4730649341289,0.663591432522345,7.24535155971625));
#9981=CARTESIAN_POINT('Ctrl Pts',(0.132960879091397,0.79722593466705,7.27319113961288));
#9982=CARTESIAN_POINT('Ctrl Pts',(-0.221169909840595,0.770191731078306,
7.30111344023989));
#9983=CARTESIAN_POINT('Ctrl Pts',(-0.510129926337539,0.631566987709629,
7.32599432900486));
#9984=CARTESIAN_POINT('Ctrl Pts',(-0.735763837282209,0.348621542769495,
7.3540721600674));
#9985=CARTESIAN_POINT('Ctrl Pts',(-0.83074585327453,-0.0641608327867673,
7.3869287659578));
#9986=CARTESIAN_POINT('Ctrl Pts',(-0.666251881204893,-0.537438189822527,
7.42461915123026));
#9987=CARTESIAN_POINT('Ctrl Pts',(-0.186253797849981,-0.839407882375731,
7.46721707138755));
#9988=CARTESIAN_POINT('Ctrl Pts',(0.379235215212093,-0.776034988224205,
7.51001044866301));
#9989=CARTESIAN_POINT('Ctrl Pts',(0.7843241358807,-0.372132898206059,7.55299798483595));
#9990=CARTESIAN_POINT('Ctrl Pts',(0.848523687541135,0.198935849878105,7.59618388556079));
#9991=CARTESIAN_POINT('Ctrl Pts',(0.575836363091698,0.632786382406762,7.63474102091317));
#9992=CARTESIAN_POINT('Ctrl Pts',(0.182120705834638,0.82172473976296,7.66860508915414));
#9993=CARTESIAN_POINT('Ctrl Pts',(-0.192836060916266,0.822151380448873,
7.69771720303896));
#9994=CARTESIAN_POINT('Ctrl Pts',(-0.531935486527566,0.658842663751575,
7.72691217814189));
#9995=CARTESIAN_POINT('Ctrl Pts',(-0.767436874667562,0.363991194653926,
7.75619251137578));
#9996=CARTESIAN_POINT('Ctrl Pts',(-0.851500538204596,-0.00484208671020629,
7.78555379321598));
#9997=CARTESIAN_POINT('Ctrl Pts',(-0.753813471543185,-0.436920652186791,
7.81990555837298));
#9998=CARTESIAN_POINT('Ctrl Pts',(-0.384264491926787,-0.807797014739186,
7.8592962103847));
#9999=CARTESIAN_POINT('Ctrl Pts',(0.204099197055569,-0.874613173770796,
7.90379252019873));
#10000=CARTESIAN_POINT('Ctrl Pts',(0.707183452191518,-0.558568943332804,
7.94845404074619));
#10001=CARTESIAN_POINT('Ctrl Pts',(0.838610010719861,-0.184049422120409,
7.97835344453705));
#10002=CARTESIAN_POINT('Ctrl Pts',(0.838635708308469,0.00449233626619855,
7.99331236500559));
#10003=CARTESIAN_POINT('Ctrl Pts',(0.733118691230247,-0.00121541092765636,
6.86520410690199));
#10004=CARTESIAN_POINT('Ctrl Pts',(0.733096176038643,0.163977229099494,
6.87831050609139));
#10005=CARTESIAN_POINT('Ctrl Pts',(0.61822085349322,0.491745228826158,6.90448596327338));
#10006=CARTESIAN_POINT('Ctrl Pts',(0.175970062539601,0.769921108293996,
6.94373227235256));
#10007=CARTESIAN_POINT('Ctrl Pts',(-0.255552194481174,0.720610916570717,
6.97641400866452));
#10008=CARTESIAN_POINT('Ctrl Pts',(-0.493113212192604,0.551270519052718,
6.99928612393978));
#10009=CARTESIAN_POINT('Ctrl Pts',(-0.599352677367421,0.425413827161342,
7.01235409532875));
#10010=CARTESIAN_POINT('Ctrl Pts',(-0.716053322126291,0.228307160798129,
7.0305039837357));
#10011=CARTESIAN_POINT('Ctrl Pts',(-0.755987795799746,-0.0402317376255194,
7.05119646804638));
#10012=CARTESIAN_POINT('Ctrl Pts',(-0.657812414621087,-0.357757242991282,
7.07733373637638));
#10013=CARTESIAN_POINT('Ctrl Pts',(-0.471441715442261,-0.591889140959248,
7.10057459246807));
#10014=CARTESIAN_POINT('Ctrl Pts',(-0.167720266372115,-0.738248710573425,
7.12672490984441));
#10015=CARTESIAN_POINT('Ctrl Pts',(0.113172505182452,-0.73814555008345,
7.14852996458262));
#10016=CARTESIAN_POINT('Ctrl Pts',(0.32139189594574,-0.665125967717377,
7.16597855239755));
#10017=CARTESIAN_POINT('Ctrl Pts',(0.508368992958891,-0.547828363309776,
7.18343278966605));
#10018=CARTESIAN_POINT('Ctrl Pts',(0.68379727163952,-0.328042392259005,
7.20526336568707));
#10019=CARTESIAN_POINT('Ctrl Pts',(0.758995968879483,0.00147100263930197,
7.23147983992185));
#10020=CARTESIAN_POINT('Ctrl Pts',(0.683845346105746,0.330894269024558,
7.25771830557115));
#10021=CARTESIAN_POINT('Ctrl Pts',(0.4494984993554,0.625611121189165,7.28690416485887));
#10022=CARTESIAN_POINT('Ctrl Pts',(0.128190915608229,0.751732271497407,
7.3132032011683));
#10023=CARTESIAN_POINT('Ctrl Pts',(-0.205740395995592,0.726211680022978,
7.33953609531371));
#10024=CARTESIAN_POINT('Ctrl Pts',(-0.47784093637727,0.595622453011025,
7.3629701633916));
#10025=CARTESIAN_POINT('Ctrl Pts',(-0.689925933091511,0.329571628023445,
7.38936942831608));
#10026=CARTESIAN_POINT('Ctrl Pts',(-0.779030370279855,-0.057949305094791,
7.42021638986164));
#10027=CARTESIAN_POINT('Ctrl Pts',(-0.624727627139914,-0.501449572002762,
7.4555452585764));
#10028=CARTESIAN_POINT('Ctrl Pts',(-0.175673176115022,-0.783757181614016,
7.4953950638941));
#10029=CARTESIAN_POINT('Ctrl Pts',(0.352351719308904,-0.724451702416669,
7.5353596505547));
#10030=CARTESIAN_POINT('Ctrl Pts',(0.729970142788671,-0.347752667481679,
7.57544876714829));
#10031=CARTESIAN_POINT('Ctrl Pts',(0.789657111879439,0.1840317456448,7.6156657596193));
#10032=CARTESIAN_POINT('Ctrl Pts',(0.535913030225253,0.58759892475464,7.65154038131291));
#10033=CARTESIAN_POINT('Ctrl Pts',(0.169902356678922,0.763219405476266,
7.68302342417015));
#10034=CARTESIAN_POINT('Ctrl Pts',(-0.178501350955049,0.763599585157561,
7.71007496388204));
#10035=CARTESIAN_POINT('Ctrl Pts',(-0.49348507045862,0.611896218217824,
7.73719675089236));
#10036=CARTESIAN_POINT('Ctrl Pts',(-0.712165255112946,0.338087476205076,
7.76438731081332));
#10037=CARTESIAN_POINT('Ctrl Pts',(-0.790218533611398,-0.00437348680934723,
7.79165189591018));
#10038=CARTESIAN_POINT('Ctrl Pts',(-0.699522824014373,-0.405524976731812,
7.82354572726495));
#10039=CARTESIAN_POINT('Ctrl Pts',(-0.356416098090345,-0.749880696062379,
7.86012337962793));
#10040=CARTESIAN_POINT('Ctrl Pts',(0.189993874214275,-0.811999190746788,
7.90144794605881));
#10041=CARTESIAN_POINT('Ctrl Pts',(0.657467882103646,-0.518362744790317,
7.94295065081735));
#10042=CARTESIAN_POINT('Ctrl Pts',(0.779720660519966,-0.170272821142141,
7.97074475069534));
#10043=CARTESIAN_POINT('Ctrl Pts',(0.779744575002708,0.00518639006840643,
7.98466570066648));
#10044=CARTESIAN_POINT('Ctrl Pts',(0.770161787666388,-0.0049051884182797,
6.91177358097206));
#10045=CARTESIAN_POINT('Ctrl Pts',(0.77013815979716,0.168451102057769,6.92552768493576));
#10046=CARTESIAN_POINT('Ctrl Pts',(0.649534215561946,0.512222733391276,
6.95298053601555));
#10047=CARTESIAN_POINT('Ctrl Pts',(0.187168277555439,0.802638877493012,
6.99399073281223));
#10048=CARTESIAN_POINT('Ctrl Pts',(-0.262198140354615,0.751064960128479,
7.02802547805165));
#10049=CARTESIAN_POINT('Ctrl Pts',(-0.508913103682435,0.575130647460083,
7.05178092432448));
#10050=CARTESIAN_POINT('Ctrl Pts',(-0.619111082011442,0.444578654305825,
7.06533603148814));
#10051=CARTESIAN_POINT('Ctrl Pts',(-0.740044687677081,0.240300892811425,
7.08414438574734));
#10052=CARTESIAN_POINT('Ctrl Pts',(-0.781206914566788,-0.0373853933734546,
7.1055381456328));
#10053=CARTESIAN_POINT('Ctrl Pts',(-0.679897669421572,-0.364897169169454,
7.13249836635836));
#10054=CARTESIAN_POINT('Ctrl Pts',(-0.488024517524781,-0.605802178567223,
7.15641268103637));
#10055=CARTESIAN_POINT('Ctrl Pts',(-0.176195068872705,-0.755957282246966,
7.18325651241199));
#10056=CARTESIAN_POINT('Ctrl Pts',(0.111348212069435,-0.755759824660184,
7.20557366213014));
#10057=CARTESIAN_POINT('Ctrl Pts',(0.324079866150574,-0.681141300007829,
7.22340028977131));
#10058=CARTESIAN_POINT('Ctrl Pts',(0.514846340621651,-0.561445486392157,
7.24120776275288));
#10059=CARTESIAN_POINT('Ctrl Pts',(0.693392023322827,-0.337618657943588,
7.26343091101724));
#10060=CARTESIAN_POINT('Ctrl Pts',(0.769635059289149,-0.00303104269807223,
7.29004601098107));
#10061=CARTESIAN_POINT('Ctrl Pts',(0.693444862893658,0.330499664199637,
7.31661153187426));
#10062=CARTESIAN_POINT('Ctrl Pts',(0.456735603111685,0.627969916924075,
7.34607308215436));
#10063=CARTESIAN_POINT('Ctrl Pts',(0.133325789120308,0.754719670744551,
7.37253732117947));
#10064=CARTESIAN_POINT('Ctrl Pts',(-0.201749074907764,0.72905336280371,
7.39895899203418));
#10065=CARTESIAN_POINT('Ctrl Pts',(-0.474093090444533,0.598239697877912,
7.42241416461049));
#10066=CARTESIAN_POINT('Ctrl Pts',(-0.685720778229502,0.332588035449833,
7.4487655384973));
#10067=CARTESIAN_POINT('Ctrl Pts',(-0.774286915001198,-0.0531887270732548,
7.47946804042779));
#10068=CARTESIAN_POINT('Ctrl Pts',(-0.620932470247468,-0.492950794309791,
7.51450072760456));
#10069=CARTESIAN_POINT('Ctrl Pts',(-0.177226274555884,-0.771445224212861,
7.55385224805798));
#10070=CARTESIAN_POINT('Ctrl Pts',(0.342041485084231,-0.712747358770181,
7.59315236551947));
#10071=CARTESIAN_POINT('Ctrl Pts',(0.711641525266257,-0.3435411547766,7.63240925035107));
#10072=CARTESIAN_POINT('Ctrl Pts',(0.769499498225703,0.175244317707386,
7.67163866408723));
#10073=CARTESIAN_POINT('Ctrl Pts',(0.522731088231096,0.567170601537302,
7.70648697733878));
#10074=CARTESIAN_POINT('Ctrl Pts',(0.168219094722662,0.737140101731971,
7.7369745868455));
#10075=CARTESIAN_POINT('Ctrl Pts',(-0.16835708474472,0.737418193432977,
7.76310610272568));
#10076=CARTESIAN_POINT('Ctrl Pts',(-0.471829280061021,0.591148177243926,
7.78923716628898));
#10077=CARTESIAN_POINT('Ctrl Pts',(-0.68198399086596,0.327873199664767,
7.81537513043843));
#10078=CARTESIAN_POINT('Ctrl Pts',(-0.756748500370122,-0.000565030967214881,
7.84151856236785));
#10079=CARTESIAN_POINT('Ctrl Pts',(-0.669865274993425,-0.38439027917607,
7.87203298976409));
#10080=CARTESIAN_POINT('Ctrl Pts',(-0.342313195892621,-0.712763775423981,
7.90692835262793));
#10081=CARTESIAN_POINT('Ctrl Pts',(0.177398463143254,-0.7716047406813,7.94622450426568));
#10082=CARTESIAN_POINT('Ctrl Pts',(0.620527880128547,-0.492889698198811,
7.98557967631099));
#10083=CARTESIAN_POINT('Ctrl Pts',(0.735934674957884,-0.163847720445079,
8.01184392471022));
#10084=CARTESIAN_POINT('Ctrl Pts',(0.735957278350781,0.00199209850848452,
8.02500167121408));
#10085=CARTESIAN_POINT('Ctrl Pts',(0.829769160098015,-0.00488434981852912,
6.91161333010028));
#10086=CARTESIAN_POINT('Ctrl Pts',(0.829743731513962,0.18168367969413,6.92641565464919));
#10087=CARTESIAN_POINT('Ctrl Pts',(0.699843619304575,0.552076534387807,
6.95599547018192));
#10088=CARTESIAN_POINT('Ctrl Pts',(0.201807308649101,0.864839644355192,
7.00016592964866));
#10089=CARTESIAN_POINT('Ctrl Pts',(-0.282182757851473,0.809306837023904,
7.03682727121008));
#10090=CARTESIAN_POINT('Ctrl Pts',(-0.547830385030607,0.619853772524046,
7.06240625604372));
#10091=CARTESIAN_POINT('Ctrl Pts',(-0.666466802209058,0.479305181004825,
7.07699970635685));
#10092=CARTESIAN_POINT('Ctrl Pts',(-0.796644113642904,0.259407192366027,
7.09724627700515));
#10093=CARTESIAN_POINT('Ctrl Pts',(-0.840912181483199,-0.039422086776628,
7.12027012001651));
#10094=CARTESIAN_POINT('Ctrl Pts',(-0.731934331083525,-0.39168152176215,
7.14926800599663));
#10095=CARTESIAN_POINT('Ctrl Pts',(-0.525629581163318,-0.650666172634783,
7.17498018991238));
#10096=CARTESIAN_POINT('Ctrl Pts',(-0.190594423194871,-0.811959054684044,
7.20382069278616));
#10097=CARTESIAN_POINT('Ctrl Pts',(0.118112171533783,-0.811717843255708,
7.22778228750397));
#10098=CARTESIAN_POINT('Ctrl Pts',(0.34634335321456,-0.731654669484967,
7.24690838696606));
#10099=CARTESIAN_POINT('Ctrl Pts',(0.550917836533123,-0.603286916074073,
7.26600558166793));
#10100=CARTESIAN_POINT('Ctrl Pts',(0.742230550690213,-0.363395535342033,
7.28982294732455));
#10101=CARTESIAN_POINT('Ctrl Pts',(0.823803964770561,-0.00519553417755166,
7.31831706475512));
#10102=CARTESIAN_POINT('Ctrl Pts',(0.742286337798943,0.351438553015085,
7.34672450759284));
#10103=CARTESIAN_POINT('Ctrl Pts',(0.489421995978955,0.6691072759963,7.37819256480912));
#10104=CARTESIAN_POINT('Ctrl Pts',(0.144523960155876,0.804171605789853,
7.40641314354085));
#10105=CARTESIAN_POINT('Ctrl Pts',(-0.212256980349852,0.77681213732754,
7.43454828405317));
#10106=CARTESIAN_POINT('Ctrl Pts',(-0.501871263134857,0.637644584928468,
7.45949448325541));
#10107=CARTESIAN_POINT('Ctrl Pts',(-0.726514202805803,0.355546311452734,
7.4874740822851));
#10108=CARTESIAN_POINT('Ctrl Pts',(-0.820312452345266,-0.0533892841775268,
7.52001935409191));
#10109=CARTESIAN_POINT('Ctrl Pts',(-0.657900019665717,-0.518447994161681,
7.55707673798875));
#10110=CARTESIAN_POINT('Ctrl Pts',(-0.189795967929553,-0.8119193538092,
7.59858280456595));
#10111=CARTESIAN_POINT('Ctrl Pts',(0.35616630218894,-0.749919823012872,
7.63990940642612));
#10112=CARTESIAN_POINT('Ctrl Pts',(0.743338323366643,-0.362709574793551,
7.68106196817871));
#10113=CARTESIAN_POINT('Ctrl Pts',(0.80346227090447,0.17923740027597,7.72204264617022));
#10114=CARTESIAN_POINT('Ctrl Pts',(0.54632793895988,0.587079715364954,7.75832537027638));
#10115=CARTESIAN_POINT('Ctrl Pts',(0.17836408415985,0.763367126788049,7.78996864240415));
#10116=CARTESIAN_POINT('Ctrl Pts',(-0.170075123139509,0.763558723590948,
7.8170221887093));
#10117=CARTESIAN_POINT('Ctrl Pts',(-0.483417494252776,0.612419263894165,
7.84400997409509));
#10118=CARTESIAN_POINT('Ctrl Pts',(-0.699782787807372,0.341192770179666,
7.87093148920761));
#10119=CARTESIAN_POINT('Ctrl Pts',(-0.776490880144409,0.00376884031652594,
7.8977917364649));
#10120=CARTESIAN_POINT('Ctrl Pts',(-0.687344347841935,-0.389454218058659,
7.9290563908098));
#10121=CARTESIAN_POINT('Ctrl Pts',(-0.352645458615756,-0.724542442309527,
7.96469323566261));
#10122=CARTESIAN_POINT('Ctrl Pts',(0.175896300401543,-0.78400788229888,
8.00465601571697));
#10123=CARTESIAN_POINT('Ctrl Pts',(0.62441514988287,-0.501460617098908,
8.04451206072658));
#10124=CARTESIAN_POINT('Ctrl Pts',(0.740592930009457,-0.169640666497113,
8.07099633783989));
#10125=CARTESIAN_POINT('Ctrl Pts',(0.740615682275994,-0.00270857004267862,
8.08424074574123));
#10126=CARTESIAN_POINT('Ctrl Pts',(0.867052181645218,-0.00120175871753932,
6.86526211624204));
#10127=CARTESIAN_POINT('Ctrl Pts',(0.867025620419448,0.193676396638986,
6.88072376693651));
#10128=CARTESIAN_POINT('Ctrl Pts',(0.731274983219511,0.581263904795406,
6.91167582009283));
#10129=CARTESIAN_POINT('Ctrl Pts',(0.208889229873121,0.909653700476453,
6.9580206776033));
#10130=CARTESIAN_POINT('Ctrl Pts',(-0.300406904913673,0.85146343699967,
6.9965998706139));
#10131=CARTESIAN_POINT('Ctrl Pts',(-0.58050096341849,0.651757693532619,
7.0235675335524));
#10132=CARTESIAN_POINT('Ctrl Pts',(-0.705698371138862,0.503443865012817,
7.03896792854912));
#10133=CARTESIAN_POINT('Ctrl Pts',(-0.843167221724989,0.27124909392191,
7.06034804595424));
#10134=CARTESIAN_POINT('Ctrl Pts',(-0.89008391300503,-0.0447685823858592,
7.08469890727413));
#10135=CARTESIAN_POINT('Ctrl Pts',(-0.774684852554919,-0.417890972125979,
7.11541335647561));
#10136=CARTESIAN_POINT('Ctrl Pts',(-0.555918291315305,-0.692620058527589,
7.14268741589426));
#10137=CARTESIAN_POINT('Ctrl Pts',(-0.200074101514066,-0.864003221456998,
7.17332192920839));
#10138=CARTESIAN_POINT('Ctrl Pts',(0.128324923138355,-0.863804881646564,
7.19881425454244));
#10139=CARTESIAN_POINT('Ctrl Pts',(0.371357425002296,-0.77855956076303,
7.21918064418244));
#10140=CARTESIAN_POINT('Ctrl Pts',(0.589346067791464,-0.641787738018295,
7.23953018657742));
#10141=CARTESIAN_POINT('Ctrl Pts',(0.793440636024401,-0.385946008896802,
7.26493567059373));
#10142=CARTESIAN_POINT('Ctrl Pts',(0.880610663516279,-0.00342731245940255,
7.29536655472608));
#10143=CARTESIAN_POINT('Ctrl Pts',(0.793503503400377,0.377874926448799,
7.32573878007044));
#10144=CARTESIAN_POINT('Ctrl Pts',(0.522907380896809,0.717918064055114,
7.35942130926836));
#10145=CARTESIAN_POINT('Ctrl Pts',(0.153358738280526,0.862712152253253,
7.38966141681963));
#10146=CARTESIAN_POINT('Ctrl Pts',(-0.229296456950172,0.83338998728552,
7.41983724018969));
#10147=CARTESIAN_POINT('Ctrl Pts',(-0.540142076806848,0.684056763209437,
7.44661190552654));
#10148=CARTESIAN_POINT('Ctrl Pts',(-0.781447811125426,0.381086249052736,
7.47666399795968));
#10149=CARTESIAN_POINT('Ctrl Pts',(-0.882294636975832,-0.0584199370281204,
7.51164340198535));
#10150=CARTESIAN_POINT('Ctrl Pts',(-0.70767939754827,-0.558645777936402,
7.55150198975409));
#10151=CARTESIAN_POINT('Ctrl Pts',(-0.203895641922302,-0.874560559164748,
7.59617469651437));
#10152=CARTESIAN_POINT('Ctrl Pts',(0.383996736306925,-0.807839822902091,
7.64067503958532));
#10153=CARTESIAN_POINT('Ctrl Pts',(0.801025471050119,-0.390801899647342,
7.6849987482111));
#10154=CARTESIAN_POINT('Ctrl Pts',(0.865780475559091,0.192944577746062,
7.72913998434886));
#10155=CARTESIAN_POINT('Ctrl Pts',(0.588848361386401,0.632155121475723,
7.76821325076472));
#10156=CARTESIAN_POINT('Ctrl Pts',(0.192692163630185,0.821932819753422,
7.80227997108));
#10157=CARTESIAN_POINT('Ctrl Pts',(-0.182308387523879,0.822124958515745,
7.83139543007317));
#10158=CARTESIAN_POINT('Ctrl Pts',(-0.51937325729508,0.659521736920761,
7.86042625847278));
#10159=CARTESIAN_POINT('Ctrl Pts',(-0.751984131238383,0.367894174259561,
7.88937101849458));
#10160=CARTESIAN_POINT('Ctrl Pts',(-0.834378810498797,0.00534130500814561,
7.91823005194813));
#10161=CARTESIAN_POINT('Ctrl Pts',(-0.738628119598523,-0.416845576119052,
7.95179753903771));
#10162=CARTESIAN_POINT('Ctrl Pts',(-0.37957617275833,-0.776169891700485,
7.99001669480089));
#10163=CARTESIAN_POINT('Ctrl Pts',(0.18648963195138,-0.839684907683195,
8.03281502748034));
#10164=CARTESIAN_POINT('Ctrl Pts',(0.665920196130032,-0.537487668578003,
8.07542274768869));
#10165=CARTESIAN_POINT('Ctrl Pts',(0.789769227401029,-0.183278618129617,
8.10368855968049));
#10166=CARTESIAN_POINT('Ctrl Pts',(0.789793474622567,-0.00537812113452141,
8.11780320149054));
#10167=CARTESIAN_POINT('Ctrl Pts',(0.853661640305302,0.00339334784518846,
6.80732253543625));
#10168=CARTESIAN_POINT('Ctrl Pts',(0.853635468008913,0.19541795114282,6.82255778504901));
#10169=CARTESIAN_POINT('Ctrl Pts',(0.719986974510146,0.577745947714341,
6.85307843059456));
#10170=CARTESIAN_POINT('Ctrl Pts',(0.202996091663939,0.9032416170388,6.89896358845432));
#10171=CARTESIAN_POINT('Ctrl Pts',(-0.303109174735908,0.845693094909515,
6.93729140028491));
#10172=CARTESIAN_POINT('Ctrl Pts',(-0.582255539424857,0.646737893808958,
6.9641625146133));
#10173=CARTESIAN_POINT('Ctrl Pts',(-0.707187570039253,0.498743335043288,
6.97952935315777));
#10174=CARTESIAN_POINT('Ctrl Pts',(-0.844496668315667,0.266850006910183,
7.00088222244567));
#10175=CARTESIAN_POINT('Ctrl Pts',(-0.891594037992852,-0.0494074690447157,
7.02524936934462));
#10176=CARTESIAN_POINT('Ctrl Pts',(-0.775864913170373,-0.423790227055181,
7.05606566088994));
#10177=CARTESIAN_POINT('Ctrl Pts',(-0.556014141834938,-0.700023509989886,
7.08348029571907));
#10178=CARTESIAN_POINT('Ctrl Pts',(-0.197442128244194,-0.872850275371536,
7.11435377694941));
#10179=CARTESIAN_POINT('Ctrl Pts',(0.134307910883221,-0.872732581079474,
7.14010240054951));
#10180=CARTESIAN_POINT('Ctrl Pts',(0.380290026930844,-0.786472573424526,
7.16071470827779));
#10181=CARTESIAN_POINT('Ctrl Pts',(0.601188873497654,-0.647894974478719,
7.18133439191931));
#10182=CARTESIAN_POINT('Ctrl Pts',(0.80843467014646,-0.388244947436199,
7.20712128927313));
#10183=CARTESIAN_POINT('Ctrl Pts',(0.897241113296386,0.00096693004960254,
7.23808404606463));
#10184=CARTESIAN_POINT('Ctrl Pts',(0.808491004798083,0.389917959096619,
7.26906263331152));
#10185=CARTESIAN_POINT('Ctrl Pts',(0.531942258526264,0.73763892882448,7.30349537884369));
#10186=CARTESIAN_POINT('Ctrl Pts',(0.153146136882341,0.886248501617647,
7.33449654477937));
#10187=CARTESIAN_POINT('Ctrl Pts',(-0.240065070170912,0.856166302038153,
7.36550226255206));
#10188=CARTESIAN_POINT('Ctrl Pts',(-0.560108122366354,0.702506159088164,
7.39306447981344));
#10189=CARTESIAN_POINT('Ctrl Pts',(-0.809177049333453,0.389950400765561,
7.42407264103054));
#10190=CARTESIAN_POINT('Ctrl Pts',(-0.913577971917155,-0.0645250182065023,
7.46024471429976));
#10191=CARTESIAN_POINT('Ctrl Pts',(-0.732789529640382,-0.583312567393491,
7.50157210267981));
#10192=CARTESIAN_POINT('Ctrl Pts',(-0.20889138072868,-0.912238145067271,
7.54804130641669));
#10193=CARTESIAN_POINT('Ctrl Pts',(0.404620472690996,-0.842920924169674,
7.59447542730139));
#10194=CARTESIAN_POINT('Ctrl Pts',(0.841321536411735,-0.406654290784301,
7.64086362524321));
#10195=CARTESIAN_POINT('Ctrl Pts',(0.909589372447933,0.206086771304483,
7.68719784696282));
#10196=CARTESIAN_POINT('Ctrl Pts',(0.618292515133597,0.668535774036831,
7.72832444946292));
#10197=CARTESIAN_POINT('Ctrl Pts',(0.200396624785897,0.868830700289083,
7.76426233212836));
#10198=CARTESIAN_POINT('Ctrl Pts',(-0.195890402329679,0.869105512774701,
7.79503036801838));
#10199=CARTESIAN_POINT('Ctrl Pts',(-0.552707853806054,0.697052799739259,
7.82575875672798));
#10200=CARTESIAN_POINT('Ctrl Pts',(-0.799378718992942,0.387911126397045,
7.85644623919681));
#10201=CARTESIAN_POINT('Ctrl Pts',(-0.886927475416378,0.00295721515884234,
7.88708853513497));
#10202=CARTESIAN_POINT('Ctrl Pts',(-0.785184349752334,-0.445993117087998,
7.92278375683408));
#10203=CARTESIAN_POINT('Ctrl Pts',(-0.402839530786299,-0.828885390140482,
7.96349431373723));
#10204=CARTESIAN_POINT('Ctrl Pts',(0.201302010936541,-0.896821923448385,
8.00917558757561));
#10205=CARTESIAN_POINT('Ctrl Pts',(0.713986287258037,-0.573914344502033,
8.05472562598296));
#10206=CARTESIAN_POINT('Ctrl Pts',(0.846713007247097,-0.194478858458525,
8.0850064631985));
#10207=CARTESIAN_POINT('Ctrl Pts',(0.846738971182356,-0.00398292970981142,
8.10012042772348));
#10208=CARTESIAN_POINT('Ctrl Pts',(0.817900488558397,0.00475133480574126,
6.79014507753449));
#10209=CARTESIAN_POINT('Ctrl Pts',(0.817875394277992,0.188866598068458,
6.80475279938448));
#10210=CARTESIAN_POINT('Ctrl Pts',(0.689784750139483,0.555422299671024,
6.8340140416451));
#10211=CARTESIAN_POINT('Ctrl Pts',(0.193435302274592,0.868118944792773,
6.87807729673241));
#10212=CARTESIAN_POINT('Ctrl Pts',(-0.293256146690176,0.812871758347855,
6.9149328617589));
#10213=CARTESIAN_POINT('Ctrl Pts',(-0.562009024419609,0.621358825924622,
6.94080240280578));
#10214=CARTESIAN_POINT('Ctrl Pts',(-0.682353384796979,0.478801116976173,
6.95560474741592));
#10215=CARTESIAN_POINT('Ctrl Pts',(-0.814675078268824,0.255341759501056,
6.97618178190882));
#10216=CARTESIAN_POINT('Ctrl Pts',(-0.860168272260483,-0.0497078330155523,
6.99968650056098));
#10217=CARTESIAN_POINT('Ctrl Pts',(-0.748436652472878,-0.411235760371946,
7.02944414274922));
#10218=CARTESIAN_POINT('Ctrl Pts',(-0.535961280579827,-0.678272766320467,
7.05594466708157));
#10219=CARTESIAN_POINT('Ctrl Pts',(-0.188978255123113,-0.845572124583574,
7.08582257562938));
#10220=CARTESIAN_POINT('Ctrl Pts',(0.13248022518062,-0.845505300794893,
7.11077362222657));
#10221=CARTESIAN_POINT('Ctrl Pts',(0.371055530451376,-0.761851985697717,
7.13076512684332));
#10222=CARTESIAN_POINT('Ctrl Pts',(0.585441233097604,-0.627371491436652,
7.15077683547094));
#10223=CARTESIAN_POINT('Ctrl Pts',(0.786808305815678,-0.375161061631681,
7.17582884965771));
#10224=CARTESIAN_POINT('Ctrl Pts',(0.87325510779514,0.00343457323490477,
7.20594902792096));
#10225=CARTESIAN_POINT('Ctrl Pts',(0.78686116127143,0.382313470509998,7.23612496849841));
#10226=CARTESIAN_POINT('Ctrl Pts',(0.517164760490624,0.721540784070928,
7.2697136876539));
#10227=CARTESIAN_POINT('Ctrl Pts',(0.147101057916398,0.86683917287086,7.30000372404372));
#10228=CARTESIAN_POINT('Ctrl Pts',(-0.237651739773033,0.837437753905466,
7.33034258187388));
#10229=CARTESIAN_POINT('Ctrl Pts',(-0.5512129818335,0.686952617632169,7.35734554941477));
#10230=CARTESIAN_POINT('Ctrl Pts',(-0.795631894615633,0.380338435114614,
7.38776877999359));
#10231=CARTESIAN_POINT('Ctrl Pts',(-0.898294846189099,-0.0662073699539118,
7.42331233504687));
#10232=CARTESIAN_POINT('Ctrl Pts',(-0.720507904090487,-0.577015468903857,
7.46400084949913));
#10233=CARTESIAN_POINT('Ctrl Pts',(-0.203663618176354,-0.901805888966958,
7.50985760554902));
#10234=CARTESIAN_POINT('Ctrl Pts',(0.403204771572536,-0.833486961268272,
7.55578804854158));
#10235=CARTESIAN_POINT('Ctrl Pts',(0.836365154142795,-0.401111707981145,
7.60178359598158));
#10236=CARTESIAN_POINT('Ctrl Pts',(0.904471271556475,0.207858603382153,
7.6478348461097));
#10237=CARTESIAN_POINT('Ctrl Pts',(0.614428615698172,0.668722267241424,
7.68881129227799));
#10238=CARTESIAN_POINT('Ctrl Pts',(0.197261178437678,0.868767690888966,
7.7246899075929));
#10239=CARTESIAN_POINT('Ctrl Pts',(-0.199005609016601,0.869111738380501,
7.7554569214687));
#10240=CARTESIAN_POINT('Ctrl Pts',(-0.556427435495044,0.696852222393774,
7.78623527481754));
#10241=CARTESIAN_POINT('Ctrl Pts',(-0.803949133824011,0.38676076397028,
7.81702187878289));
#10242=CARTESIAN_POINT('Ctrl Pts',(-0.891995003933998,-5.28792355482503E-5,
7.84781415673619));
#10243=CARTESIAN_POINT('Ctrl Pts',(-0.789679403174556,-0.4519291484846,
7.88374203453794));
#10244=CARTESIAN_POINT('Ctrl Pts',(-0.404226672020434,-0.838247889347281,
7.9248014076827));
#10245=CARTESIAN_POINT('Ctrl Pts',(0.206521632311494,-0.907164419165389,
7.97098703818337));
#10246=CARTESIAN_POINT('Ctrl Pts',(0.726215048173051,-0.580160328067018,
8.01714652643371));
#10247=CARTESIAN_POINT('Ctrl Pts',(0.86119627917958,-0.194707506801938,
8.04791285500075));
#10248=CARTESIAN_POINT('Ctrl Pts',(0.861222672429394,-0.00106172137465173,
8.0632767294446));
#10249=CARTESIAN_POINT('Ctrl Pts',(0.799992192036797,0.00474896193479852,
6.79014422086044));
#10250=CARTESIAN_POINT('Ctrl Pts',(0.799967638550529,0.184896450338747,
6.80443713908974));
#10251=CARTESIAN_POINT('Ctrl Pts',(0.674670361705441,0.543455008309391,
6.8330594352144));
#10252=CARTESIAN_POINT('Ctrl Pts',(0.189034209544693,0.849439608053688,
6.87617354971506));
#10253=CARTESIAN_POINT('Ctrl Pts',(-0.287258299249701,0.795379885058583,
6.91224027998794));
#10254=CARTESIAN_POINT('Ctrl Pts',(-0.550325497980241,0.607926215999118,
6.93756224237155));
#10255=CARTESIAN_POINT('Ctrl Pts',(-0.668135787638992,0.468370262290034,
6.95205278987894));
#10256=CARTESIAN_POINT('Ctrl Pts',(-0.797681515793003,0.249601245171223,
6.97219797725517));
#10257=CARTESIAN_POINT('Ctrl Pts',(-0.842241289744138,-0.0491002547813337,
6.99521334099182));
#10258=CARTESIAN_POINT('Ctrl Pts',(-0.732812122296168,-0.403197173369283,
7.02435916833342));
#10259=CARTESIAN_POINT('Ctrl Pts',(-0.524668382980495,-0.664806008100517,
7.0503201318013));
#10260=CARTESIAN_POINT('Ctrl Pts',(-0.184652568425117,-0.828760962866216,
7.07959861118036));
#10261=CARTESIAN_POINT('Ctrl Pts',(0.130453782933179,-0.82870656943649,
7.10405631433573));
#10262=CARTESIAN_POINT('Ctrl Pts',(0.364375751582702,-0.746687575144636,
7.12365775087804));
#10263=CARTESIAN_POINT('Ctrl Pts',(0.574616121324387,-0.614810215974657,
7.14328235821488));
#10264=CARTESIAN_POINT('Ctrl Pts',(0.772150732123964,-0.367420603086453,
7.16785616546509));
#10265=CARTESIAN_POINT('Ctrl Pts',(0.856997117769862,0.00408861547259015,
7.19741267271575));
#10266=CARTESIAN_POINT('Ctrl Pts',(0.772201652552023,0.376032772307348,
7.22703591400899));
#10267=CARTESIAN_POINT('Ctrl Pts',(0.507351873091063,0.709199534687239,
7.26002305113266));
#10268=CARTESIAN_POINT('Ctrl Pts',(0.143736848284574,0.852002078379093,
7.28978615651597));
#10269=CARTESIAN_POINT('Ctrl Pts',(-0.234502546384647,0.823108658745492,
7.31961111148852));
#10270=CARTESIAN_POINT('Ctrl Pts',(-0.542883282495364,0.675129422402413,
7.34616719094667));
#10271=CARTESIAN_POINT('Ctrl Pts',(-0.783396359273759,0.37345029211527,
7.3761020331664));
#10272=CARTESIAN_POINT('Ctrl Pts',(-0.884489493081995,-0.0661466723839558,
7.41109301032321));
#10273=CARTESIAN_POINT('Ctrl Pts',(-0.709418296017906,-0.569369739308696,
7.45117535759087));
#10274=CARTESIAN_POINT('Ctrl Pts',(-0.19989068769657,-0.889667511851702,
7.49638689971083));
#10275=CARTESIAN_POINT('Ctrl Pts',(0.398973895326053,-0.822339305277361,
7.54171055210185));
#10276=CARTESIAN_POINT('Ctrl Pts',(0.826865587387622,-0.395358142551438,
7.58713932258037));
#10277=CARTESIAN_POINT('Ctrl Pts',(0.894293657405342,0.206666783144423,
7.6326658525427));
#10278=CARTESIAN_POINT('Ctrl Pts',(0.607352590357856,0.662764035303079,
7.67321405418637));
#10279=CARTESIAN_POINT('Ctrl Pts',(0.194215191945802,0.860916697467946,
7.70874703376387));
#10280=CARTESIAN_POINT('Ctrl Pts',(-0.198496552114366,0.86128604965953,
7.7392380606388));
#10281=CARTESIAN_POINT('Ctrl Pts',(-0.552965374281963,0.690483866395827,
7.76976084505319));
#10282=CARTESIAN_POINT('Ctrl Pts',(-0.798625493103115,0.382774108679761,
7.80031292414605));
#10283=CARTESIAN_POINT('Ctrl Pts',(-0.886090514398701,-0.00135276288038935,
7.83089169974969));
#10284=CARTESIAN_POINT('Ctrl Pts',(-0.784450923473031,-0.450417071001065,
7.86659566812776));
#10285=CARTESIAN_POINT('Ctrl Pts',(-0.401130832210515,-0.834733160113732,
7.90743505712395));
#10286=CARTESIAN_POINT('Ctrl Pts',(0.206987829997999,-0.903462960885791,
7.95342319362056));
#10287=CARTESIAN_POINT('Ctrl Pts',(0.725081242328631,-0.57760276120548,
7.99943459556092));
#10288=CARTESIAN_POINT('Ctrl Pts',(0.859845779758374,-0.192969267412252,
8.03013735189051));
#10289=CARTESIAN_POINT('Ctrl Pts',(0.85987212861708,0.000350822954683268,
8.04547538565828));
#10290=CARTESIAN_POINT('',(0.740013321878819,-3.30221092258282E-6,6.84996753665487));
#10291=CARTESIAN_POINT('',(0.86002906121511,-2.8436073730086E-6,6.85013896332608));
#10292=CARTESIAN_POINT('Ctrl Pts',(0.740023219291072,-5.77198260618599E-6,
6.85002034628079));
#10293=CARTESIAN_POINT('Ctrl Pts',(0.740021358405138,-2.10300419701926E-5,
6.85039822499709));
#10294=CARTESIAN_POINT('Ctrl Pts',(0.740023024222631,-3.62850179820163E-5,
6.85077606240544));
#10295=CARTESIAN_POINT('Ctrl Pts',(0.740028231502145,-5.1534688844035E-5,
6.85115380766388));
#10296=CARTESIAN_POINT('Ctrl Pts',(0.740085053936413,-0.00021794085503002,
6.85527580746438));
#10297=CARTESIAN_POINT('Ctrl Pts',(0.740561847799387,-0.00038290723370555,
6.85936598291913));
#10298=CARTESIAN_POINT('Ctrl Pts',(0.741474476273296,-0.00054348152203615,
6.86335924813516));
#10299=CARTESIAN_POINT('Ctrl Pts',(0.742233180141228,-0.000676973229921408,
6.86667900623136));
#10300=CARTESIAN_POINT('Ctrl Pts',(0.743293477943993,-0.000807438902367973,
6.86993201105744));
#10301=CARTESIAN_POINT('Ctrl Pts',(0.744631277735025,-0.000933850565882489,
6.87308796691842));
#10302=CARTESIAN_POINT('Ctrl Pts',(0.746754426168902,-0.00113447156105222,
6.8780966108041));
#10303=CARTESIAN_POINT('Ctrl Pts',(0.749546546792157,-0.00132241308026135,
6.88279723847818));
#10304=CARTESIAN_POINT('Ctrl Pts',(0.752899116929639,-0.00149305386639579,
6.88707335410488));
#10305=CARTESIAN_POINT('Ctrl Pts',(0.754360743054021,-0.00156744844150423,
6.88893762004252));
#10306=CARTESIAN_POINT('Ctrl Pts',(0.755929524328344,-0.00163854499625076,
6.89072092401184));
#10307=CARTESIAN_POINT('Ctrl Pts',(0.757598887046534,-0.00170586425030808,
6.89241168757878));
#10308=CARTESIAN_POINT('Ctrl Pts',(0.761394051663765,-0.001858909270586,
6.89625550533956));
#10309=CARTESIAN_POINT('Ctrl Pts',(0.765657159823746,-0.00199058430570913,
6.89957326466661));
#10310=CARTESIAN_POINT('Ctrl Pts',(0.770297905279784,-0.00209437976410097,
6.90224220648893));
#10311=CARTESIAN_POINT('Ctrl Pts',(0.771480718348967,-0.00212083470024662,
6.9029224548021));
#10312=CARTESIAN_POINT('Ctrl Pts',(0.772688227465772,-0.00214546614515498,
6.90356035260593));
#10313=CARTESIAN_POINT('Ctrl Pts',(0.773919225517153,-0.00216813570411822,
6.90415338933386));
#10314=CARTESIAN_POINT('Ctrl Pts',(0.774849981021487,-0.00218527611856664,
6.90460178338141));
#10315=CARTESIAN_POINT('Ctrl Pts',(0.77579416755915,-0.00220129455406626,
6.90502452541544));
#10316=CARTESIAN_POINT('Ctrl Pts',(0.77675073101501,-0.0022162186817045,
6.90542159869653));
#10317=CARTESIAN_POINT('Ctrl Pts',(0.781727100262787,-0.0022938590822172,
6.90748730929108));
#10318=CARTESIAN_POINT('Ctrl Pts',(0.786971413210206,-0.00234111121487575,
6.90883536506399));
#10319=CARTESIAN_POINT('Ctrl Pts',(0.792325599468412,-0.00236147596166846,
6.90948862972605));
#10320=CARTESIAN_POINT('Ctrl Pts',(0.794699452788802,-0.00237050495682504,
6.90977826374556));
#10321=CARTESIAN_POINT('Ctrl Pts',(0.797095176688634,-0.00237419920632471,
6.90993065281261));
#10322=CARTESIAN_POINT('Ctrl Pts',(0.799499433912905,-0.00237262251695804,
6.90994459926205));
#10323=CARTESIAN_POINT('Ctrl Pts',(0.804934689322609,-0.00236905812737313,
6.90997612771666));
#10324=CARTESIAN_POINT('Ctrl Pts',(0.810341856817132,-0.00233882740457025,
6.909303140357));
#10325=CARTESIAN_POINT('Ctrl Pts',(0.815566649891691,-0.00228184659800146,
6.90793064851273));
#10326=CARTESIAN_POINT('Ctrl Pts',(0.817867829031793,-0.00225675028479036,
6.90732615574968));
#10327=CARTESIAN_POINT('Ctrl Pts',(0.820133625359067,-0.00222640701590779,
6.90658530716917));
#10328=CARTESIAN_POINT('Ctrl Pts',(0.822349983198305,-0.00219053233431339,
6.90570540025299));
#10329=CARTESIAN_POINT('Ctrl Pts',(0.823602413960143,-0.00217026008675276,
6.90520817797694));
#10330=CARTESIAN_POINT('Ctrl Pts',(0.82483494206673,-0.00214828094937227,
6.90466814014931));
#10331=CARTESIAN_POINT('Ctrl Pts',(0.826045257442232,-0.00212456411533838,
6.90408538174413));
#10332=CARTESIAN_POINT('Ctrl Pts',(0.830894037694746,-0.0020295494449117,
6.90175072789755));
#10333=CARTESIAN_POINT('Ctrl Pts',(0.835388487964696,-0.00190698894305515,
6.89873407321304));
#10334=CARTESIAN_POINT('Ctrl Pts',(0.839441071831611,-0.00176396566847474,
6.89516397873058));
#10335=CARTESIAN_POINT('Ctrl Pts',(0.840235771719969,-0.001735919221054,
6.89446389360469));
#10336=CARTESIAN_POINT('Ctrl Pts',(0.841013384724027,-0.00170707348974732,
6.89374239738474));
#10337=CARTESIAN_POINT('Ctrl Pts',(0.841773092391,-0.00167746545197683,
6.89300029288931));
#10338=CARTESIAN_POINT('Ctrl Pts',(0.845672921400161,-0.00152547766822612,
6.88919082674212));
#10339=CARTESIAN_POINT('Ctrl Pts',(0.84905256830136,-0.00135568308239744,
6.88489142900407));
#10340=CARTESIAN_POINT('Ctrl Pts',(0.851819498119605,-0.00117319323714043,
6.88022796254556));
#10341=CARTESIAN_POINT('Ctrl Pts',(0.853029466194191,-0.00109339110943874,
6.87818864608206));
#10342=CARTESIAN_POINT('Ctrl Pts',(0.854121791492832,-0.0010111142513845,
6.8760792357492));
#10343=CARTESIAN_POINT('Ctrl Pts',(0.855085995445545,-0.0009266211082642,
6.87390868773667));
#10344=CARTESIAN_POINT('Ctrl Pts',(0.85659857140088,-0.000794074154567515,
6.87050368330332));
#10345=CARTESIAN_POINT('Ctrl Pts',(0.85778271855372,-0.000657301396693565,
6.86697912957925));
#10346=CARTESIAN_POINT('Ctrl Pts',(0.858606344933536,-0.000517333545493498,
6.86337295784898));
#10347=CARTESIAN_POINT('Ctrl Pts',(0.859509064743485,-0.000363924481468129,
6.8594204828691));
#10348=CARTESIAN_POINT('Ctrl Pts',(0.859979039725546,-0.000206633239390191,
6.85536955609449));
#10349=CARTESIAN_POINT('Ctrl Pts',(0.860033114959129,-4.77911640563713E-5,
6.85128419258908));
#10350=CARTESIAN_POINT('Ctrl Pts',(0.860038121181873,-3.30857479617889E-5,
6.85090597434861));
#10351=CARTESIAN_POINT('Ctrl Pts',(0.860039548467556,-1.83741767728084E-5,
6.85052764184536));
#10352=CARTESIAN_POINT('Ctrl Pts',(0.860037413159089,-3.65835365705083E-6,
6.85014924671004));
#10353=CARTESIAN_POINT('',(0.799999353205575,0.00474549275567414,6.79018795858619));
#10354=CARTESIAN_POINT('Origin',(0.8,3.02639196116122E-20,6.85));
#10355=CARTESIAN_POINT('',(0.859872007312157,8.03685277434799E-7,8.04544761499495));
#10356=CARTESIAN_POINT('Ctrl Pts',(0.799992192036797,0.00474896193479852,
6.79014422086044));
#10357=CARTESIAN_POINT('Ctrl Pts',(0.799967638550529,0.184896450338747,
6.80443713908974));
#10358=CARTESIAN_POINT('Ctrl Pts',(0.674670361705441,0.543455008309391,
6.8330594352144));
#10359=CARTESIAN_POINT('Ctrl Pts',(0.189034209544693,0.849439608053688,
6.87617354971506));
#10360=CARTESIAN_POINT('Ctrl Pts',(-0.287258299249701,0.795379885058583,
6.91224027998794));
#10361=CARTESIAN_POINT('Ctrl Pts',(-0.550325497980241,0.607926215999118,
6.93756224237155));
#10362=CARTESIAN_POINT('Ctrl Pts',(-0.668135787638992,0.468370262290034,
6.95205278987894));
#10363=CARTESIAN_POINT('Ctrl Pts',(-0.797681515793003,0.249601245171223,
6.97219797725517));
#10364=CARTESIAN_POINT('Ctrl Pts',(-0.842241289744138,-0.0491002547813337,
6.99521334099182));
#10365=CARTESIAN_POINT('Ctrl Pts',(-0.732812122296168,-0.403197173369283,
7.02435916833342));
#10366=CARTESIAN_POINT('Ctrl Pts',(-0.524668382980495,-0.664806008100517,
7.0503201318013));
#10367=CARTESIAN_POINT('Ctrl Pts',(-0.184652568425117,-0.828760962866216,
7.07959861118036));
#10368=CARTESIAN_POINT('Ctrl Pts',(0.130453782933179,-0.82870656943649,
7.10405631433573));
#10369=CARTESIAN_POINT('Ctrl Pts',(0.364375751582702,-0.746687575144636,
7.12365775087804));
#10370=CARTESIAN_POINT('Ctrl Pts',(0.574616121324387,-0.614810215974657,
7.14328235821488));
#10371=CARTESIAN_POINT('Ctrl Pts',(0.772150732123964,-0.367420603086453,
7.16785616546509));
#10372=CARTESIAN_POINT('Ctrl Pts',(0.856997117769862,0.00408861547259015,
7.19741267271575));
#10373=CARTESIAN_POINT('Ctrl Pts',(0.772201652552023,0.376032772307348,
7.22703591400899));
#10374=CARTESIAN_POINT('Ctrl Pts',(0.507351873091063,0.709199534687239,
7.26002305113266));
#10375=CARTESIAN_POINT('Ctrl Pts',(0.143736848284574,0.852002078379093,
7.28978615651597));
#10376=CARTESIAN_POINT('Ctrl Pts',(-0.234502546384647,0.823108658745492,
7.31961111148852));
#10377=CARTESIAN_POINT('Ctrl Pts',(-0.542883282495364,0.675129422402413,
7.34616719094667));
#10378=CARTESIAN_POINT('Ctrl Pts',(-0.783396359273759,0.37345029211527,
7.3761020331664));
#10379=CARTESIAN_POINT('Ctrl Pts',(-0.884489493081995,-0.0661466723839558,
7.41109301032321));
#10380=CARTESIAN_POINT('Ctrl Pts',(-0.709418296017906,-0.569369739308696,
7.45117535759087));
#10381=CARTESIAN_POINT('Ctrl Pts',(-0.19989068769657,-0.889667511851702,
7.49638689971083));
#10382=CARTESIAN_POINT('Ctrl Pts',(0.398973895326053,-0.822339305277361,
7.54171055210185));
#10383=CARTESIAN_POINT('Ctrl Pts',(0.826865587387622,-0.395358142551438,
7.58713932258037));
#10384=CARTESIAN_POINT('Ctrl Pts',(0.894293657405342,0.206666783144423,
7.6326658525427));
#10385=CARTESIAN_POINT('Ctrl Pts',(0.607352590357856,0.662764035303079,
7.67321405418637));
#10386=CARTESIAN_POINT('Ctrl Pts',(0.194215191945802,0.860916697467946,
7.70874703376387));
#10387=CARTESIAN_POINT('Ctrl Pts',(-0.198496552114366,0.86128604965953,
7.7392380606388));
#10388=CARTESIAN_POINT('Ctrl Pts',(-0.552965374281963,0.690483866395827,
7.76976084505319));
#10389=CARTESIAN_POINT('Ctrl Pts',(-0.798625493103115,0.382774108679761,
7.80031292414605));
#10390=CARTESIAN_POINT('Ctrl Pts',(-0.886090514398701,-0.00135276288038935,
7.83089169974969));
#10391=CARTESIAN_POINT('Ctrl Pts',(-0.784450923473031,-0.450417071001065,
7.86659566812776));
#10392=CARTESIAN_POINT('Ctrl Pts',(-0.401130832210515,-0.834733160113732,
7.90743505712395));
#10393=CARTESIAN_POINT('Ctrl Pts',(0.206987829997999,-0.903462960885791,
7.95342319362056));
#10394=CARTESIAN_POINT('Ctrl Pts',(0.724977015357669,-0.577668315834745,
7.99942533925898));
#10395=CARTESIAN_POINT('Ctrl Pts',(0.859764427178652,-0.19320138704919,
8.03011882209587));
#10396=CARTESIAN_POINT('Ctrl Pts',(0.859872007312956,8.05120031746468E-7,
8.04544761510878));
#10397=CARTESIAN_POINT('Ctrl Pts',(0.859872007312157,8.03685277532201E-7,
8.04544761499494));
#10398=CARTESIAN_POINT('Ctrl Pts',(0.859872039269663,5.81957034837644E-5,
8.04545216851661));
#10399=CARTESIAN_POINT('Ctrl Pts',(0.859872065291453,0.000115587812293562,
8.0454567220371));
#10400=CARTESIAN_POINT('Ctrl Pts',(0.859872085377142,0.000172980010638188,
8.04546127555641));
#10401=CARTESIAN_POINT('Origin',(0.8,3.02639196116122E-20,6.85));
#10402=CARTESIAN_POINT('Origin',(0.8,-3.5,6.85));
#10403=CARTESIAN_POINT('Origin',(0.8,0.,6.85));
#10404=CARTESIAN_POINT('',(0.74,-3.5,6.85));
#10405=CARTESIAN_POINT('',(0.74,-3.5,6.85));
#10406=CARTESIAN_POINT('Origin',(0.8,-3.5,6.85));
#10407=CARTESIAN_POINT('Origin',(0.8,0.,6.85));
#10408=CARTESIAN_POINT('',(0.8,0.,6.85));
#10409=CARTESIAN_POINT('Origin',(0.8,-3.5,6.85));
#10410=CARTESIAN_POINT('Origin',(0.8,3.02639196116122E-20,6.85));
#12708=UNCERTAINTY_MEASURE_WITH_UNIT(LENGTH_MEASURE(0.001),#12780,
'DISTANCE_ACCURACY_VALUE',
'Maximum model space distance between geometric entities at asserted c
onnectivities');
#12739=UNCERTAINTY_MEASURE_WITH_UNIT(LENGTH_MEASURE(0.001),#12780,
'DISTANCE_ACCURACY_VALUE',
'Maximum model space distance between geometric entities at asserted c
onnectivities');
#12748=(
GEOMETRIC_REPRESENTATION_CONTEXT(3)
GLOBAL_UNCERTAINTY_ASSIGNED_CONTEXT((#12708))
GLOBAL_UNIT_ASSIGNED_CONTEXT((#12780,#12782,#12783))
REPRESENTATION_CONTEXT('','3D')
);
#12779=(
GEOMETRIC_REPRESENTATION_CONTEXT(3)
GLOBAL_UNCERTAINTY_ASSIGNED_CONTEXT((#12739))
GLOBAL_UNIT_ASSIGNED_CONTEXT((#12780,#12782,#12783))
REPRESENTATION_CONTEXT('','3D')
);
#12780=(
LENGTH_UNIT()
NAMED_UNIT(*)
SI_UNIT(.CENTI.,.METRE.)
);
#12782=(
NAMED_UNIT(*)
PLANE_ANGLE_UNIT()
SI_UNIT($,.RADIAN.)
);
#12783=(
NAMED_UNIT(*)
SI_UNIT($,.STERADIAN.)
SOLID_ANGLE_UNIT()
);
#12792=SHAPE_DEFINITION_REPRESENTATION(#12831,#12931);
#12831=PRODUCT_DEFINITION_SHAPE('',$,#12971);
#12931=SHAPE_REPRESENTATION('',(#6692),#12748);
#12962=PRODUCT_DEFINITION_CONTEXT('part definition',#13081,'design');
#12971=PRODUCT_DEFINITION('Installed torsion spring',
'Installed torsion spring',#13010,#12962);
#13010=PRODUCT_DEFINITION_FORMATION('',$,#13091);
#13081=APPLICATION_CONTEXT(
'Core Data for Automotive Mechanical Design Process');
#13082=PRODUCT_CONTEXT('part definition',#13081,'mechanical');
#13091=PRODUCT('Installed torsion spring','Installed torsion spring',
'Installed torsion spring',(#13082));
#13178=COLOUR_RGB('Grey',0.48,0.52,0.57);
#13179=FILL_AREA_STYLE_COLOUR('',#13178);
#13180=FILL_AREA_STYLE('',(#13179));
#13181=SURFACE_STYLE_FILL_AREA(#13180);
#13182=SURFACE_SIDE_STYLE('',(#13181));
#13183=SURFACE_STYLE_USAGE(.BOTH.,#13182);
#13184=PRESENTATION_STYLE_ASSIGNMENT((#13183));
ENDSEC;
END-ISO-10303-21;
